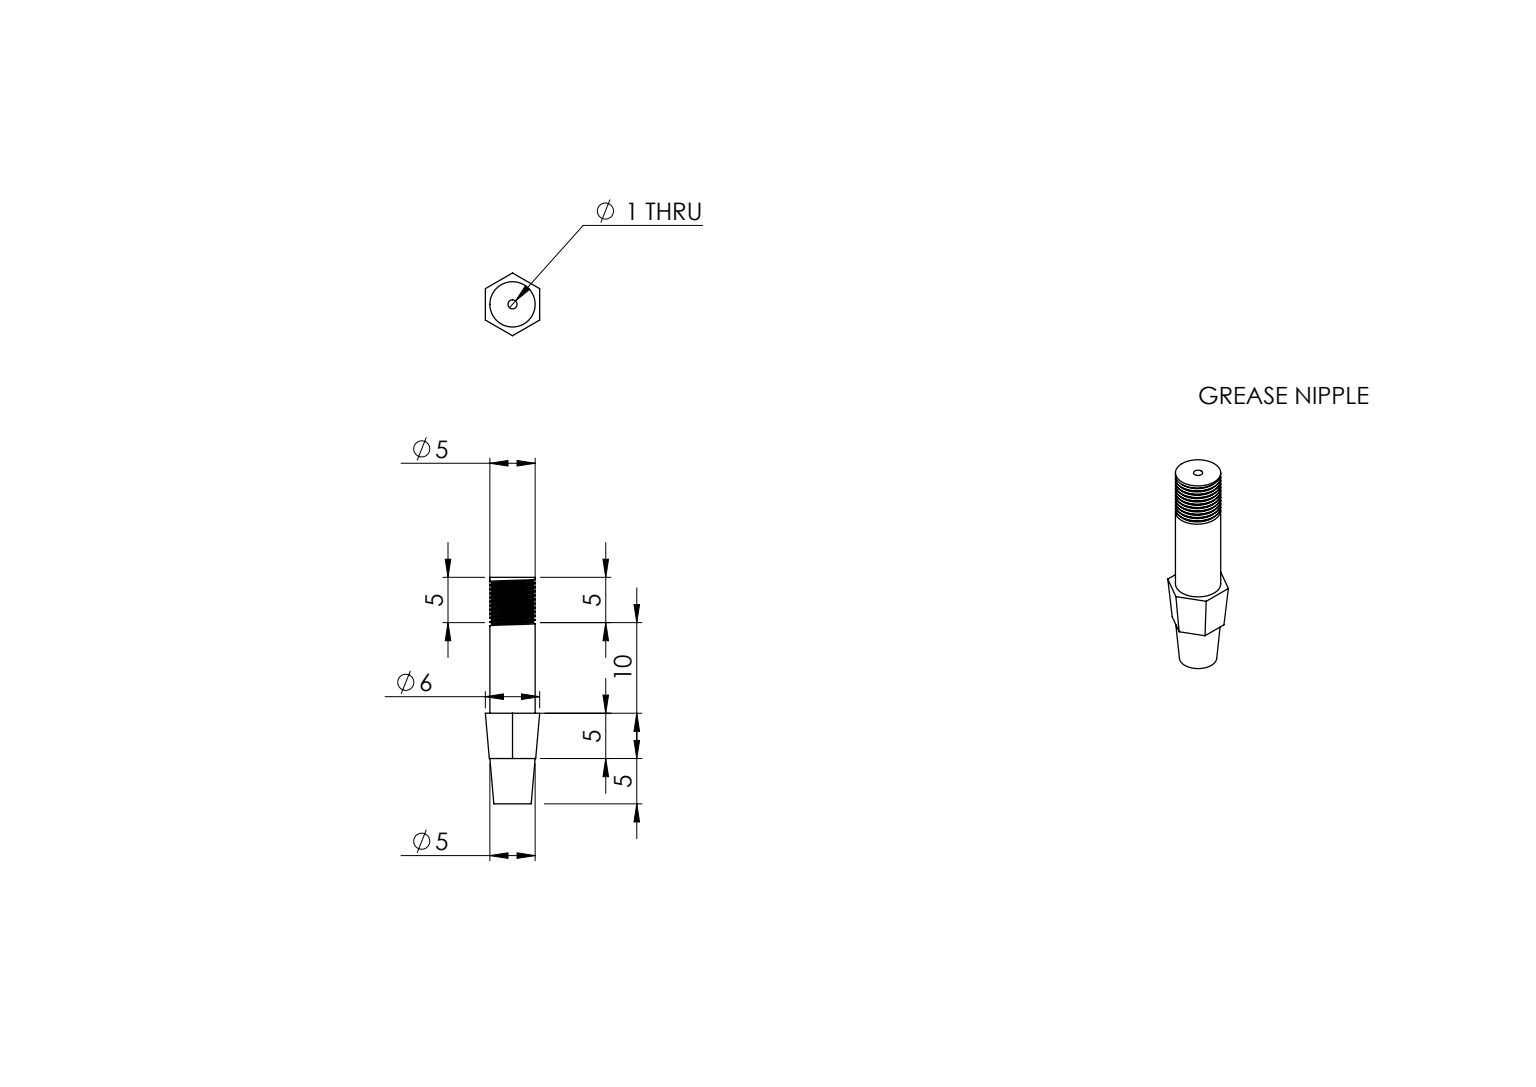
ISO-10303-21;
HEADER;
FILE_DESCRIPTION (('STEP AP214'),
    '1' );
FILE_NAME ('grease nipple.step',
    '2026-10-24T15:06:47',
    ( '' ),
    ( '' ),
    'SwSTEP 2.0',
    'SolidWorks 2026',
    '' );
FILE_SCHEMA (( 'AUTOMOTIVE_DESIGN' ));
ENDSEC;

DATA;
#3=CARTESIAN_POINT ( 'NONE',  ( 4.786228327491940187E-16, -2.728124999385483473, 2.605501347177161087 ) ) ;
#7=CARTESIAN_POINT ( 'NONE',  ( 2.256430356249999658, -2.578124999385483118, -1.302750673588581432 ) ) ;
#11=LINE ( 'NONE', #3942, #5600 ) ;
#16=CARTESIAN_POINT ( 'NONE',  ( 1.128215178125001161, -4.153124999385482852, 1.954126010382870815 ) ) ;
#20=CARTESIAN_POINT ( 'NONE',  ( 1.249999999999999334, -1.050000000000000044, -2.165063509461096825 ) ) ;
#21=CARTESIAN_POINT ( 'NONE',  ( 1.128215178124999607, -3.103124999385482585, -1.954126010382871259 ) ) ;
#25=CARTESIAN_POINT ( 'NONE',  ( 1.250000000000001110, -2.043749998770965970, 2.165063509461096380 ) ) ;
#27=CARTESIAN_POINT ( 'NONE',  ( 1.249999999999999334, -0.9937499987709658145, -2.165063509461096825 ) ) ;
#28=CARTESIAN_POINT ( 'NONE',  ( -2.499999999999999112, -3.112499999999999822, 1.443375672974065882 ) ) ;
#30=CARTESIAN_POINT ( 'NONE',  ( 4.786228327491941173E-16, -3.178124999385482763, 2.605501347177161087 ) ) ;
#31=ORIENTED_EDGE ( 'NONE', *, *, #3987, .F. ) ;
#34=ORIENTED_EDGE ( 'NONE', *, *, #3622, .T. ) ;
#37=CARTESIAN_POINT ( 'NONE',  ( 1.034219503716432668E-14, -3.656249998770965792, -2.500000000000000000 ) ) ;
#40=AXIS2_PLACEMENT_3D ( 'NONE', #3682, #8497, #6028 ) ;
#42=EDGE_CURVE ( 'NONE', #3838, #8637, #9238, .T. ) ;
#46=CARTESIAN_POINT ( 'NONE',  ( -2.256430356249999214, -3.365624999385482319, 1.302750673588581876 ) ) ;
#54=CARTESIAN_POINT ( 'NONE',  ( 3.061616997868383141E-16, 0.000000000000000000, 2.500000000000000000 ) ) ;
#55=CARTESIAN_POINT ( 'NONE',  ( -1.128215178124998497, -3.665624999385482585, 1.954126010382872147 ) ) ;
#57=ORIENTED_EDGE ( 'NONE', *, *, #3072, .T. ) ;
#60=CARTESIAN_POINT ( 'NONE',  ( -2.256430356250000102, -1.940624999385482941, 0.000000000000000000 ) ) ;
#77=CARTESIAN_POINT ( 'NONE',  ( 9.877377282685029372E-16, -1.237499999999999600, 2.500000000000000000 ) ) ;
#78=CARTESIAN_POINT ( 'NONE',  ( 2.256430356250000546, -4.565624999385482496, 1.302750673588579877 ) ) ;
#79=CARTESIAN_POINT ( 'NONE',  ( -4.357666448243394824E-15, -2.531249998770965348, 2.500000000000000000 ) ) ;
#83=CARTESIAN_POINT ( 'NONE',  ( -1.250000000000000222, -4.518749998770965171, -2.165063509461096825 ) ) ;
#88=LINE ( 'NONE', #2497, #4362 ) ;
#89=CARTESIAN_POINT ( 'NONE',  ( 2.256430356249999658, -3.928124999385482319, -1.302750673588581432 ) ) ;
#95=CARTESIAN_POINT ( 'NONE',  ( -2.499999999999999112, -3.506249998770964993, 1.443375672974065882 ) ) ;
#98=ORIENTED_EDGE ( 'NONE', *, *, #7857, .T. ) ;
#99=CARTESIAN_POINT ( 'NONE',  ( 0.000000000000000000, 0.000000000000000000, 0.000000000000000000 ) ) ;
#102=CARTESIAN_POINT ( 'NONE',  ( -2.256430356250000102, -0.1781249993854829572, -1.302750673588580321 ) ) ;
#103=EDGE_CURVE ( 'NONE', #3372, #2494, #7434, .T. ) ;
#104=FACE_OUTER_BOUND ( 'NONE', #9219, .T. ) ;
#110=CARTESIAN_POINT ( 'NONE',  ( -1.128215178124998497, -4.115624999385482319, 1.954126010382872147 ) ) ;
#112=EDGE_LOOP ( 'NONE', ( #9331, #6596, #10060, #487 ) ) ;
#114=CARTESIAN_POINT ( 'NONE',  ( -1.128215178124998497, -3.665624999385482585, 1.954126010382872147 ) ) ;
#121=EDGE_CURVE ( 'NONE', #3756, #7561, #4966, .T. ) ;
#125=ORIENTED_EDGE ( 'NONE', *, *, #7390, .T. ) ;
#127=CARTESIAN_POINT ( 'NONE',  ( 1.250000000000001110, -5.193749998770964993, 2.165063509461096380 ) ) ;
#130=CARTESIAN_POINT ( 'NONE',  ( -2.256430356250000102, -4.303124999385482319, 0.000000000000000000 ) ) ;
#135=CARTESIAN_POINT ( 'NONE',  ( -1.249999999999998224, -4.368749998770964815, 2.165063509461097713 ) ) ;
#138=FACE_OUTER_BOUND ( 'NONE', #6423, .T. ) ;
#141=CARTESIAN_POINT ( 'NONE',  ( -1.128215178125000273, -3.815624999385482941, -1.954126010382871259 ) ) ;
#147=CARTESIAN_POINT ( 'NONE',  ( 1.250000000000001110, -3.843749998770965348, 2.165063509461096380 ) ) ;
#149=EDGE_LOOP ( 'NONE', ( #7106, #3257, #2787, #8826 ) ) ;
#159=CARTESIAN_POINT ( 'NONE',  ( 1.034219503716432668E-14, -4.612500000000000711, -2.500000000000000000 ) ) ;
#160=ORIENTED_EDGE ( 'NONE', *, *, #2379, .T. ) ;
#161=CARTESIAN_POINT ( 'NONE',  ( -2.256430356249999214, -4.153124999385482852, 1.302750673588581876 ) ) ;
#166=CARTESIAN_POINT ( 'NONE',  ( 6.307557144418638510E-17, -20.00000000000000000, -2.958985580760425727 ) ) ;
#167=CARTESIAN_POINT ( 'NONE',  ( 1.250000000000001110, -3.449999999999999289, 2.165063509461096380 ) ) ;
#170=CARTESIAN_POINT ( 'NONE',  ( 1.249999999999999334, -1.443749998770965881, -2.165063509461096825 ) ) ;
#171=CARTESIAN_POINT ( 'NONE',  ( 2.500000000000000000, -4.218749998770966236, -3.061616997868383141E-16 ) ) ;
#172=EDGE_CURVE ( 'NONE', #957, #2983, #5656, .T. ) ;
#173=CARTESIAN_POINT ( 'NONE',  ( -1.128215178125000273, -4.828124999385481786, -1.954126010382871259 ) ) ;
#178=CARTESIAN_POINT ( 'NONE',  ( -1.250000000000000222, -3.618749998770965259, -2.165063509461096825 ) ) ;
#181=EDGE_CURVE ( 'NONE', #471, #3838, #8521, .T. ) ;
#186=CARTESIAN_POINT ( 'NONE',  ( 1.128215178125001161, -4.490624999385482319, 1.954126010382870815 ) ) ;
#191=EDGE_CURVE ( 'NONE', #3656, #1900, #9595, .T. ) ;
#192=PLANE ( 'NONE',  #10324 ) ;
#193=ORIENTED_EDGE ( 'NONE', *, *, #8350, .T. ) ;
#197=CARTESIAN_POINT ( 'NONE',  ( 6.123233995736709336E-17, -25.00000000000000000, 0.4999999999999953371 ) ) ;
#206=CARTESIAN_POINT ( 'NONE',  ( -0.6698729810778081273, -2.157596189432334111, 2.499999999999999112 ) ) ;
#208=CARTESIAN_POINT ( 'NONE',  ( 2.256430356250000546, -4.003124999385482496, 1.302750673588579877 ) ) ;
#211=VECTOR ( 'NONE', #9822, 1000.000000000000000 ) ;
#213=CARTESIAN_POINT ( 'NONE',  ( 2.500000000000000000, -0.6187499987709659255, -3.061616997868383141E-16 ) ) ;
#222=CARTESIAN_POINT ( 'NONE',  ( 2.500000000000000444, -2.456249998770965615, 1.443375672974063439 ) ) ;
#228=CARTESIAN_POINT ( 'NONE',  ( 1.249999999999999334, -5.043749998770965526, -2.165063509461096825 ) ) ;
#230=ORIENTED_EDGE ( 'NONE', *, *, #6289, .F. ) ;
#234=( BOUNDED_CURVE ( )  B_SPLINE_CURVE ( 1, ( #10186, #707 ),
 .UNSPECIFIED., .F., .F. ) 
 B_SPLINE_CURVE_WITH_KNOTS ( ( 2, 2 ),
 ( 0.000000000000000000, 1.000000000000000000 ),
 .UNSPECIFIED. ) 
 CURVE ( )  GEOMETRIC_REPRESENTATION_ITEM ( )  RATIONAL_B_SPLINE_CURVE ( ( 0.9401538480137057174, 0.9401538480137057174 ) ) 
 REPRESENTATION_ITEM ( '' )  );
#238=DIRECTION ( 'NONE',  ( 0.000000000000000000, 0.000000000000000000, -1.000000000000000000 ) ) ;
#239=DIRECTION ( 'NONE',  ( 0.000000000000000000, -1.000000000000000000, 0.000000000000000000 ) ) ;
#253=CARTESIAN_POINT ( 'NONE',  ( -1.250000000000000222, -2.324999999999999734, -2.165063509461096825 ) ) ;
#254=VECTOR ( 'NONE', #2667, 1000.000000000000000 ) ;
#256=CARTESIAN_POINT ( 'NONE',  ( -2.256430356250000546, -5.114265350234221685, -0.8212662131217605133 ) ) ;
#257=SURFACE_STYLE_USAGE ( .BOTH. , #8210 ) ;
#263=ADVANCED_FACE ( 'NONE', ( #4540 ), #1407, .T. ) ;
#270=DIRECTION ( 'NONE',  ( 0.000000000000000000, -1.000000000000000000, 0.000000000000000000 ) ) ;
#273=CARTESIAN_POINT ( 'NONE',  ( 0.000000000000000000, 0.000000000000000000, -2.500000000000000000 ) ) ;
#276=CARTESIAN_POINT ( 'NONE',  ( 4.786228327491941173E-16, -0.5906249993854828517, 2.605501347177161087 ) ) ;
#280=CYLINDRICAL_SURFACE ( 'NONE', #8136, 0.4999999999999953371 ) ;
#287=CARTESIAN_POINT ( 'NONE',  ( 3.061616997868383141E-16, 0.000000000000000000, 2.500000000000000000 ) ) ;
#289=( BOUNDED_CURVE ( )  B_SPLINE_CURVE ( 2, ( #364, #2666, #6794, #9834, #213, #3555, #2617, #5222, #2774 ),
 .UNSPECIFIED., .F., .F. ) 
 B_SPLINE_CURVE_WITH_KNOTS ( ( 3, 2, 2, 2, 3 ),
 ( 0.02083333333333333218, 0.02777777777777777624, 0.04166666666666666435, 0.05555555555555555247, 0.06250000000000000000 ),
 .UNSPECIFIED. ) 
 CURVE ( )  GEOMETRIC_REPRESENTATION_ITEM ( )  RATIONAL_B_SPLINE_CURVE ( ( 0.9330127018922194093, 0.9330127018922194093, 1.000000000000000000, 0.8660254037844387076, 1.000000000000000000, 0.8660254037844387076, 1.000000000000000000, 0.9330127018922194093, 0.9330127018922194093 ) ) 
 REPRESENTATION_ITEM ( '' )  );
#290=ORIENTED_EDGE ( 'NONE', *, *, #2409, .F. ) ;
#293=CARTESIAN_POINT ( 'NONE',  ( -0.6698729810778054627, -2.101346188203299548, 2.500000000000000000 ) ) ;
#308=ORIENTED_EDGE ( 'NONE', *, *, #1549, .F. ) ;
#309=CARTESIAN_POINT ( 'NONE',  ( 5.302876193624534821E-16, -0.3375000000000000222, 2.886751345948128655 ) ) ;
#311=CARTESIAN_POINT ( 'NONE',  ( -2.499999999999999112, -2.662500000000000089, 1.443375672974065882 ) ) ;
#312=CARTESIAN_POINT ( 'NONE',  ( -2.256430356250000102, -0.2906249993854829183, -1.302750673588580321 ) ) ;
#323=CARTESIAN_POINT ( 'NONE',  ( -2.256430356249998770, -5.165624999385483029, 1.302750673588581876 ) ) ;
#329=CARTESIAN_POINT ( 'NONE',  ( -1.128215178124998497, -0.6281249993854828295, 1.954126010382872147 ) ) ;
#338=CARTESIAN_POINT ( 'NONE',  ( 0.000000000000000000, -15.00000000000000000, -3.464101615137755275 ) ) ;
#344=DIRECTION ( 'NONE',  ( 0.000000000000000000, 0.000000000000000000, -1.000000000000000000 ) ) ;
#350=( BOUNDED_CURVE ( )  B_SPLINE_CURVE ( 2, ( #1905, #2558, #5099, #3338, #9762, #1029, #2603, #8299, #3536 ),
 .UNSPECIFIED., .F., .T. ) 
 B_SPLINE_CURVE_WITH_KNOTS ( ( 3, 2, 2, 2, 3 ),
 ( 0.8125000000000000000, 0.8194444444444444198, 0.8333333333333333703, 0.8472222222222222099, 0.8541666666666667407 ),
 .UNSPECIFIED. ) 
 CURVE ( )  GEOMETRIC_REPRESENTATION_ITEM ( )  RATIONAL_B_SPLINE_CURVE ( ( 0.9330127018922194093, 0.9330127018922194093, 1.000000000000000000, 0.8660254037844387076, 1.000000000000000000, 0.8660254037844387076, 1.000000000000000000, 0.9330127018922187432, 0.9330127018922192983 ) ) 
 REPRESENTATION_ITEM ( '' )  );
#352=DIRECTION ( 'NONE',  ( 0.000000000000000000, -1.000000000000000000, 0.000000000000000000 ) ) ;
#353=ADVANCED_FACE ( 'NONE', ( #2833 ), #3833, .T. ) ;
#354=CYLINDRICAL_SURFACE ( 'NONE', #9119, 2.500000000000000000 ) ;
#357=CARTESIAN_POINT ( 'NONE',  ( -2.499999999999999112, -4.856249998770965526, 1.443375672974065882 ) ) ;
#359=CARTESIAN_POINT ( 'NONE',  ( 2.500000000000000000, -2.887500000000000178, -1.443375672974064994 ) ) ;
#364=CARTESIAN_POINT ( 'NONE',  ( -3.486133158594716510E-16, -0.5062499987709657701, -2.500000000000000000 ) ) ;
#372=CARTESIAN_POINT ( 'NONE',  ( 2.256430356250000102, -0.3656249993854829294, -2.763330213280484622E-16 ) ) ;
#381=CARTESIAN_POINT ( 'NONE',  ( 2.256430356250000102, -0.9281249993854827629, -2.763330213280484622E-16 ) ) ;
#384=FACE_OUTER_BOUND ( 'NONE', #8353, .T. ) ;
#386=CARTESIAN_POINT ( 'NONE',  ( -4.357666448243394824E-15, -2.137500000000000178, 2.500000000000000000 ) ) ;
#391=FACE_OUTER_BOUND ( 'NONE', #6159, .T. ) ;
#397=CARTESIAN_POINT ( 'NONE',  ( -3.000000000000000888, -15.00000000000000000, 1.732050807568878525 ) ) ;
#400=EDGE_LOOP ( 'NONE', ( #6468, #2775, #6027, #9450 ) ) ;
#404=CARTESIAN_POINT ( 'NONE',  ( -0.6698729810778054627, -0.3575961894323341772, 2.500000000000000000 ) ) ;
#407=AXIS2_PLACEMENT_3D ( 'NONE', #3351, #3996, #8023 ) ;
#409=EDGE_LOOP ( 'NONE', ( #1063, #2661, #6306, #7148 ) ) ;
#410=CARTESIAN_POINT ( 'NONE',  ( -2.500000000000000000, -0.9375000000000000000, -1.443375672974064106 ) ) ;
#413=CARTESIAN_POINT ( 'NONE',  ( 4.786228327491941173E-16, -0.5906249993854828517, 2.605501347177161087 ) ) ;
#416=ORIENTED_EDGE ( 'NONE', *, *, #4589, .F. ) ;
#418=LINE ( 'NONE', #2620, #6815 ) ;
#425=CARTESIAN_POINT ( 'NONE',  ( 2.256430356250000102, -0.8156249993854828295, -2.763330213280484622E-16 ) ) ;
#433=CARTESIAN_POINT ( 'NONE',  ( 2.256430356250000546, -2.315624999385482496, 1.302750673588579877 ) ) ;
#450=ADVANCED_FACE ( 'NONE', ( #1363 ), #4557, .T. ) ;
#455=CARTESIAN_POINT ( 'NONE',  ( 9.877377282685029372E-16, -0.7312499987709657479, 2.500000000000000000 ) ) ;
#457=CARTESIAN_POINT ( 'NONE',  ( -0.6698729810778069060, -4.086153809338631149, -2.500000000000000000 ) ) ;
#465=CARTESIAN_POINT ( 'NONE',  ( -1.249999999999998224, -1.274999999999999911, 2.165063509461097713 ) ) ;
#468=CARTESIAN_POINT ( 'NONE',  ( -2.256430356249999214, -2.015624999385482674, 1.302750673588581876 ) ) ;
#471=VERTEX_POINT ( 'NONE', #5661 ) ;
#477=CARTESIAN_POINT ( 'NONE',  ( 1.128215178125001161, -0.4406249993854829405, 1.954126010382870815 ) ) ;
#478=CARTESIAN_POINT ( 'NONE',  ( -1.250000000000000222, -4.124999999999999112, -2.165063509461096825 ) ) ;
#480=CARTESIAN_POINT ( 'NONE',  ( 0.6698729810778075722, -1.611153809338631282, 2.499999999999999556 ) ) ;
#487=ORIENTED_EDGE ( 'NONE', *, *, #10255, .F. ) ;
#489=CARTESIAN_POINT ( 'NONE',  ( 2.256430356250000102, -2.278124999385482852, -2.763330213280484622E-16 ) ) ;
#494=CARTESIAN_POINT ( 'NONE',  ( 1.034219503716432668E-14, -4.556249998770965703, -2.500000000000000000 ) ) ;
#502=CARTESIAN_POINT ( 'NONE',  ( 4.996790860652426159E-15, -2.306249998770965259, -2.500000000000000000 ) ) ;
#506=CARTESIAN_POINT ( 'NONE',  ( 2.256430356249999658, -1.228124999385483029, -1.302750673588581432 ) ) ;
#512=EDGE_CURVE ( 'NONE', #9561, #3286, #7220, .T. ) ;
#515=ORIENTED_EDGE ( 'NONE', *, *, #3140, .T. ) ;
#516=ADVANCED_FACE ( 'NONE', ( #8750 ), #3205, .T. ) ;
#520=CARTESIAN_POINT ( 'NONE',  ( 1.250000000000001110, -2.549999999999999822, 2.165063509461096380 ) ) ;
#524=CARTESIAN_POINT ( 'NONE',  ( 1.249999999999999334, -3.750000000000000000, -2.165063509461096825 ) ) ;
#525=CARTESIAN_POINT ( 'NONE',  ( 1.128215178124999607, -0.8531249993854828073, -1.954126010382871259 ) ) ;
#534=CARTESIAN_POINT ( 'NONE',  ( -2.256430356250000102, -1.078124999385482896, -1.302750673588580321 ) ) ;
#545=CARTESIAN_POINT ( 'NONE',  ( 1.128215178125001161, -2.803124999385482319, 1.954126010382870815 ) ) ;
#551=CARTESIAN_POINT ( 'NONE',  ( 1.128215178124999607, -1.303124999385482985, -1.954126010382871259 ) ) ;
#554=CARTESIAN_POINT ( 'NONE',  ( -1.767625397874844694E-16, -0.9562499987709658367, -2.886751345948128655 ) ) ;
#555=DIRECTION ( 'NONE',  ( 0.000000000000000000, 0.000000000000000000, -1.000000000000000000 ) ) ;
#559=CARTESIAN_POINT ( 'NONE',  ( 2.500000000000000444, -4.312499999999999112, 1.443375672974063439 ) ) ;
#560=CARTESIAN_POINT ( 'NONE',  ( -2.256430356250000102, -2.390624999385482674, 0.000000000000000000 ) ) ;
#562=EDGE_CURVE ( 'NONE', #8637, #5955, #6441, .T. ) ;
#571=CARTESIAN_POINT ( 'NONE',  ( -2.500000000000000000, -2.250000000000000000, 0.000000000000000000 ) ) ;
#572=PRODUCT_CONTEXT ( 'NONE', #2270, 'mechanical' ) ;
#575=( BOUNDED_CURVE ( )  B_SPLINE_CURVE ( 2, ( #6071, #8326, #1930, #9321, #2035, #1365, #5230 ),
 .UNSPECIFIED., .F., .F. ) 
 B_SPLINE_CURVE_WITH_KNOTS ( ( 3, 2, 2, 3 ),
 ( 0.8958333333333333703, 0.9027777777777777901, 0.9166666666666666297, 0.9258784757798345089 ),
 .UNSPECIFIED. ) 
 CURVE ( )  GEOMETRIC_REPRESENTATION_ITEM ( )  RATIONAL_B_SPLINE_CURVE ( ( 0.9330127018922192983, 0.9330127018922198534, 1.000000000000000000, 0.8660254037844387076, 1.000000000000000000, 0.9111413147426927761, 0.9401537210011674528 ) ) 
 REPRESENTATION_ITEM ( '' )  );
#576=CARTESIAN_POINT ( 'NONE',  ( -1.595409442497313560E-16, -2.615624999385482319, -2.605501347177161087 ) ) ;
#581=CARTESIAN_POINT ( 'NONE',  ( -2.500000000000000000, -3.131249998770965881, -1.443375672974064106 ) ) ;
#586=CARTESIAN_POINT ( 'NONE',  ( 2.256430356250000546, -0.4031249993854829627, 1.302750673588579877 ) ) ;
#599=CARTESIAN_POINT ( 'NONE',  ( -1.595409442497313560E-16, -4.865624999385482319, -2.605501347177161087 ) ) ;
#602=CARTESIAN_POINT ( 'NONE',  ( 0.6698729810778075722, -0.3174038105676657562, 2.499999999999999556 ) ) ;
#603=AXIS2_PLACEMENT_3D ( 'NONE', #2574, #5908, #1150 ) ;
#604=CARTESIAN_POINT ( 'NONE',  ( 2.256430356250000546, -1.415624999385482807, 1.302750673588579877 ) ) ;
#607=CARTESIAN_POINT ( 'NONE',  ( -2.500000000000000000, -0.3937499987709658922, 0.000000000000000000 ) ) ;
#609=DIRECTION ( 'NONE',  ( 0.8660254037844384856, -0.000000000000000000, 0.5000000000000003331 ) ) ;
#610=LINE ( 'NONE', #5438, #3877 ) ;
#611=CARTESIAN_POINT ( 'NONE',  ( -2.256430356250000102, -1.040624999385483029, 0.000000000000000000 ) ) ;
#617=CARTESIAN_POINT ( 'NONE',  ( -1.250000000000000222, -4.068749998770965881, -2.165063509461096825 ) ) ;
#621=VECTOR ( 'NONE', #847, 1000.000000000000000 ) ;
#625=CARTESIAN_POINT ( 'NONE',  ( -2.500000000000000000, -4.537500000000000533, -1.443375672974064106 ) ) ;
#627=CARTESIAN_POINT ( 'NONE',  ( 1.128215178124999607, -3.103124999385482585, -1.954126010382871259 ) ) ;
#635=CARTESIAN_POINT ( 'NONE',  ( -1.128215178125000273, -0.2156249993854829905, -1.954126010382871259 ) ) ;
#640=CARTESIAN_POINT ( 'NONE',  ( -2.256430356250000102, -2.840624999385482852, 0.000000000000000000 ) ) ;
#641=( BOUNDED_CURVE ( )  B_SPLINE_CURVE ( 2, ( #5478, #4466, #4837, #8031, #171, #6505, #3954, #5728, #2381 ),
 .UNSPECIFIED., .F., .T. ) 
 B_SPLINE_CURVE_WITH_KNOTS ( ( 3, 2, 2, 2, 3 ),
 ( 0.6875000000000000000, 0.6944444444444444198, 0.7083333333333333703, 0.7222222222222222099, 0.7291666666666667407 ),
 .UNSPECIFIED. ) 
 CURVE ( )  GEOMETRIC_REPRESENTATION_ITEM ( )  RATIONAL_B_SPLINE_CURVE ( ( 0.9330127018922194093, 0.9330127018922194093, 1.000000000000000000, 0.8660254037844387076, 1.000000000000000000, 0.8660254037844387076, 1.000000000000000000, 0.9330127018922187432, 0.9330127018922192983 ) ) 
 REPRESENTATION_ITEM ( '' )  );
#652=CARTESIAN_POINT ( 'NONE',  ( 2.256430356250000546, -3.215624999385482408, 1.302750673588579877 ) ) ;
#654=ORIENTED_EDGE ( 'NONE', *, *, #4623, .F. ) ;
#658=CARTESIAN_POINT ( 'NONE',  ( -2.256430356250000102, -2.540624999385482141, -1.302750673588580321 ) ) ;
#660=CARTESIAN_POINT ( 'NONE',  ( 0.000000000000000000, -15.00000000000000000, 0.000000000000000000 ) ) ;
#661=CARTESIAN_POINT ( 'NONE',  ( 2.500000000000000000, -2.381249998770965437, -1.443375672974064994 ) ) ;
#666=CARTESIAN_POINT ( 'NONE',  ( 1.128215178125001161, -0.8906249993854828961, 1.954126010382870815 ) ) ;
#680=CARTESIAN_POINT ( 'NONE',  ( 1.128215178124999607, -1.753124999385482718, -1.954126010382871259 ) ) ;
#687=DIRECTION ( 'NONE',  ( 0.000000000000000000, -1.000000000000000000, 0.000000000000000000 ) ) ;
#689=CARTESIAN_POINT ( 'NONE',  ( 1.128215178124999607, -0.2906249993854829738, -1.954126010382871259 ) ) ;
#690=CARTESIAN_POINT ( 'NONE',  ( 9.877377282685029372E-16, -3.431249998770965259, 2.500000000000000000 ) ) ;
#692=ORIENTED_EDGE ( 'NONE', *, *, #9777, .F. ) ;
#693=CARTESIAN_POINT ( 'NONE',  ( -2.256430356249999214, -1.003124999385482718, 1.302750673588581876 ) ) ;
#702=( BOUNDED_CURVE ( )  B_SPLINE_CURVE ( 2, ( #9940, #9054, #4392, #6590, #2719, #1873, #6743, #7577, #5907 ),
 .UNSPECIFIED., .F., .T. ) 
 B_SPLINE_CURVE_WITH_KNOTS ( ( 3, 2, 2, 2, 3 ),
 ( 0.1458333333333333426, 0.1527777777777777901, 0.1666666666666666574, 0.1805555555555555525, 0.1875000000000000000 ),
 .UNSPECIFIED. ) 
 CURVE ( )  GEOMETRIC_REPRESENTATION_ITEM ( )  RATIONAL_B_SPLINE_CURVE ( ( 0.9330127018922194093, 0.9330127018922194093, 1.000000000000000000, 0.8660254037844387076, 1.000000000000000000, 0.8660254037844387076, 1.000000000000000000, 0.9330127018922194093, 0.9330127018922194093 ) ) 
 REPRESENTATION_ITEM ( '' )  );
#703=CARTESIAN_POINT ( 'NONE',  ( -2.256430356250000102, -4.340624999385482852, -1.302750673588580321 ) ) ;
#705=ADVANCED_FACE ( 'NONE', ( #3545 ), #354, .T. ) ;
#707=CARTESIAN_POINT ( 'NONE',  ( -1.915118561403101438, -5.394273269507307234, -1.606960141313192203 ) ) ;
#708=CARTESIAN_POINT ( 'NONE',  ( -2.256430356250000102, -1.640624999385482896, -1.302750673588580321 ) ) ;
#711=AXIS2_PLACEMENT_3D ( 'NONE', #5088, #4310, #7495 ) ;
#713=CARTESIAN_POINT ( 'NONE',  ( -2.499999999999999556, -2.156249998770965348, 1.443375672974065882 ) ) ;
#716=CARTESIAN_POINT ( 'NONE',  ( -2.500000000000000000, -3.187500000000000000, -1.443375672974064106 ) ) ;
#719=CARTESIAN_POINT ( 'NONE',  ( 1.128215178125001161, -0.4406249993854829405, 1.954126010382870815 ) ) ;
#720=CIRCLE ( 'NONE', #4552, 2.500000000000000444 ) ;
#721=ORIENTED_EDGE ( 'NONE', *, *, #4686, .T. ) ;
#722=EDGE_CURVE ( 'NONE', #8554, #8603, #2756, .T. ) ;
#733=CARTESIAN_POINT ( 'NONE',  ( 2.500000000000000000, -4.237499999999999822, -1.443375672974064994 ) ) ;
#735=CARTESIAN_POINT ( 'NONE',  ( 1.128215178124999607, -4.903124999385481964, -1.954126010382871259 ) ) ;
#736=CARTESIAN_POINT ( 'NONE',  ( 0.000000000000000000, 0.000000000000000000, 0.000000000000000000 ) ) ;
#742=DIRECTION ( 'NONE',  ( -0.08715574274765837404, -0.9961946980917455452, 0.000000000000000000 ) ) ;
#743=CARTESIAN_POINT ( 'NONE',  ( 4.786228327491940187E-16, -4.078124999385482674, 2.605501347177161087 ) ) ;
#747=CARTESIAN_POINT ( 'NONE',  ( -2.256430356249999214, -1.903124999385482852, 1.302750673588581876 ) ) ;
#757=CARTESIAN_POINT ( 'NONE',  ( -2.256430356250000990, -5.226765388979074167, -0.8212675591186288093 ) ) ;
#764=CARTESIAN_POINT ( 'NONE',  ( -1.128215178125000273, -2.578124999385482674, -1.954126010382871259 ) ) ;
#768=CARTESIAN_POINT ( 'NONE',  ( 9.877377282685029372E-16, -1.687499999999999778, 2.500000000000000000 ) ) ;
#769=CARTESIAN_POINT ( 'NONE',  ( -2.499999999999999556, -3.056249998770965259, 1.443375672974065882 ) ) ;
#770=ORIENTED_EDGE ( 'NONE', *, *, #2670, .T. ) ;
#773=CARTESIAN_POINT ( 'NONE',  ( -0.6698729810778020211, -3.242403810567665357, -2.500000000000002665 ) ) ;
#774=FACE_OUTER_BOUND ( 'NONE', #10183, .T. ) ;
#775=CARTESIAN_POINT ( 'NONE',  ( 1.128215178124999607, -3.440624999385482496, -1.954126010382871259 ) ) ;
#778=ORIENTED_EDGE ( 'NONE', *, *, #7478, .F. ) ;
#785=CARTESIAN_POINT ( 'NONE',  ( -1.345399338949505808, -5.026709289312093709, -2.285932919781461958 ) ) ;
#788=CARTESIAN_POINT ( 'NONE',  ( -1.595409442497313560E-16, -4.415624999385482141, -2.605501347177161087 ) ) ;
#791=UNCERTAINTY_MEASURE_WITH_UNIT (LENGTH_MEASURE( 1.000000000000000082E-05 ), #10331, 'distance_accuracy_value', 'NONE');
#799=CARTESIAN_POINT ( 'NONE',  ( -1.595409442497313560E-16, -3.853124999385482585, -2.605501347177161087 ) ) ;
#801=CARTESIAN_POINT ( 'NONE',  ( 2.256430356250000546, -2.203124999385482674, 1.302750673588579877 ) ) ;
#806=CARTESIAN_POINT ( 'NONE',  ( -2.256430356250000102, -0.1406249993854829794, 0.000000000000000000 ) ) ;
#809=CARTESIAN_POINT ( 'NONE',  ( 0.000000000000000000, 0.000000000000000000, 0.000000000000000000 ) ) ;
#815=CARTESIAN_POINT ( 'NONE',  ( 2.256430356249999658, -4.490624999385482319, -1.302750673588581432 ) ) ;
#821=AXIS2_PLACEMENT_3D ( 'NONE', #7498, #239, #4948 ) ;
#822=CARTESIAN_POINT ( 'NONE',  ( 2.500000000000000000, -1.481249998770965970, -1.443375672974064994 ) ) ;
#824=DIRECTION ( 'NONE',  ( 0.000000000000000000, 0.000000000000000000, -1.000000000000000000 ) ) ;
#826=CARTESIAN_POINT ( 'NONE',  ( 2.256430356250000102, -4.415624999385482141, -2.763330213280484622E-16 ) ) ;
#829=CARTESIAN_POINT ( 'NONE',  ( 0.000000000000000000, -25.00000000000000000, -2.062556682370379590 ) ) ;
#830=CARTESIAN_POINT ( 'NONE',  ( 0.000000000000000000, 0.000000000000000000, 0.000000000000000000 ) ) ;
#835=CARTESIAN_POINT ( 'NONE',  ( -1.249999999999998224, -4.875000000000000000, 2.165063509461097713 ) ) ;
#838=CARTESIAN_POINT ( 'NONE',  ( -1.128215178125000273, -3.928124999385483207, -1.954126010382871259 ) ) ;
#843=EDGE_CURVE ( 'NONE', #1838, #1383, #2583, .T. ) ;
#847=DIRECTION ( 'NONE',  ( 0.000000000000000000, -1.000000000000000000, 0.000000000000000000 ) ) ;
#848=CARTESIAN_POINT ( 'NONE',  ( 1.128215178124999607, -3.440624999385482496, -1.954126010382871259 ) ) ;
#850=ADVANCED_FACE ( 'NONE', ( #5431, #7830 ), #2335, .F. ) ;
#852=CARTESIAN_POINT ( 'NONE',  ( 2.256430356250000102, -2.615624999385482763, -2.763330213280484622E-16 ) ) ;
#856=CARTESIAN_POINT ( 'NONE',  ( 1.034219503716432668E-14, -3.206249998770966059, -2.500000000000000000 ) ) ;
#859=( BOUNDED_CURVE ( )  B_SPLINE_CURVE ( 2, ( #959, #2579, #170, #5072, #8963, #4976, #4196, #480, #6128 ),
 .UNSPECIFIED., .F., .F. ) 
 B_SPLINE_CURVE_WITH_KNOTS ( ( 3, 2, 2, 2, 3 ),
 ( 0.1875000000000000000, 0.1944444444444444475, 0.2083333333333333426, 0.2222222222222222099, 0.2291666666666666574 ),
 .UNSPECIFIED. ) 
 CURVE ( )  GEOMETRIC_REPRESENTATION_ITEM ( )  RATIONAL_B_SPLINE_CURVE ( ( 0.9330127018922194093, 0.9330127018922194093, 1.000000000000000000, 0.8660254037844387076, 1.000000000000000000, 0.8660254037844387076, 1.000000000000000000, 0.9330127018922194093, 0.9330127018922194093 ) ) 
 REPRESENTATION_ITEM ( '' )  );
#865=APPLICATION_CONTEXT ( 'automotive_design' ) ;
#867=CARTESIAN_POINT ( 'NONE',  ( 1.128215178125001161, -5.053124999385482319, 1.954126010382870815 ) ) ;
#871=CARTESIAN_POINT ( 'NONE',  ( -1.249999999999998224, -2.568749998770965437, 2.165063509461097713 ) ) ;
#876=CARTESIAN_POINT ( 'NONE',  ( -2.256430356249999214, -3.703124999385482674, 1.302750673588581876 ) ) ;
#880=DIRECTION ( 'NONE',  ( 0.000000000000000000, -1.000000000000000000, 0.000000000000000000 ) ) ;
#883=VECTOR ( 'NONE', #5087, 1000.000000000000114 ) ;
#889=CARTESIAN_POINT ( 'NONE',  ( -1.128215178124998497, -5.128124999385482496, 1.954126010382872147 ) ) ;
#897=CARTESIAN_POINT ( 'NONE',  ( 2.256430356250000546, -3.553124999385482763, 1.302750673588579877 ) ) ;
#899=CARTESIAN_POINT ( 'NONE',  ( 2.256430356250000546, -4.453124999385482674, 1.302750673588579877 ) ) ;
#914=EDGE_CURVE ( 'NONE', #3286, #6080, #4178, .T. ) ;
#916=CARTESIAN_POINT ( 'NONE',  ( 2.256430356250000546, -5.015624999385481786, 1.302750673588579877 ) ) ;
#920=( BOUNDED_CURVE ( )  B_SPLINE_CURVE ( 2, ( #8344, #2554, #4366, #6572, #1021, #8932, #147, #3529, #4218 ),
 .UNSPECIFIED., .F., .T. ) 
 B_SPLINE_CURVE_WITH_KNOTS ( ( 3, 2, 2, 2, 3 ),
 ( 0.6041666666666667407, 0.6111111111111111605, 0.6250000000000000000, 0.6388888888888888395, 0.6458333333333333703 ),
 .UNSPECIFIED. ) 
 CURVE ( )  GEOMETRIC_REPRESENTATION_ITEM ( )  RATIONAL_B_SPLINE_CURVE ( ( 0.9330127018922192983, 0.9330127018922198534, 1.000000000000000000, 0.8660254037844387076, 1.000000000000000000, 0.8660254037844387076, 1.000000000000000000, 0.9330127018922187432, 0.9330127018922192983 ) ) 
 REPRESENTATION_ITEM ( '' )  );
#921=CARTESIAN_POINT ( 'NONE',  ( 2.500000000000000000, -4.631249998770965881, -1.443375672974064994 ) ) ;
#923=CYLINDRICAL_SURFACE ( 'NONE', #5111, 2.500000000000000000 ) ;
#926=CARTESIAN_POINT ( 'NONE',  ( 1.128215178125001161, -4.040624999385483029, 1.954126010382870815 ) ) ;
#929=AXIS2_PLACEMENT_3D ( 'NONE', #6755, #5824, #3568 ) ;
#935=DIRECTION ( 'NONE',  ( 0.000000000000000000, 0.000000000000000000, -1.000000000000000000 ) ) ;
#946=CARTESIAN_POINT ( 'NONE',  ( -2.256430356249998770, -4.153124999385482852, 1.302750673588581876 ) ) ;
#947=ORIENTED_EDGE ( 'NONE', *, *, #3571, .F. ) ;
#948=CARTESIAN_POINT ( 'NONE',  ( -1.595409442497313560E-16, -3.403124999385483296, -2.605501347177161087 ) ) ;
#949=FACE_OUTER_BOUND ( 'NONE', #8574, .T. ) ;
#955=LINE ( 'NONE', #7185, #3544 ) ;
#957=VERTEX_POINT ( 'NONE', #3323 ) ;
#959=CARTESIAN_POINT ( 'NONE',  ( -3.486133158594716510E-16, -1.406249998770965570, -2.500000000000000000 ) ) ;
#962=CARTESIAN_POINT ( 'NONE',  ( -2.256430356249998770, -3.815624999385482941, 1.302750673588581876 ) ) ;
#968=CARTESIAN_POINT ( 'NONE',  ( 2.500000000000000444, -5.156249998770965348, 1.443375672974063439 ) ) ;
#970=ORIENTED_EDGE ( 'NONE', *, *, #3832, .F. ) ;
#971=DIRECTION ( 'NONE',  ( 0.000000000000000000, -1.000000000000000000, 0.000000000000000000 ) ) ;
#974=( BOUNDED_CURVE ( )  B_SPLINE_CURVE ( 2, ( #9222, #7089, #10068, #5429, #4578, #10240, #10294, #2227, #2112, #8722, #4521, #9456, #7714, #1386, #9281, #8618, #6314, #2966, #3849, #2905, #5480, #1442, #7773, #3073, #3126, #4635, #5309, #1542, #551, #2282, #3744, #604, #8504, #7828, #9508, #3901, #3024, #708, #4736, #3802, #6985, #1334, #6927, #10128, #8671, #10187, #6872, #1494, #6200, #6256, #9398, #6145, #9343, #2332, #6089, #2172, #5371, #8561, #4690, #5531, #7930, #658, #764, #7038, #7875, #5580, #2581, #6362, #8869, #4057, #9745, #5774, #4786, #6463, #3956, #4107, #21, #8768, #1784, #3319, #7193, #5731, #9650, #2537, #7983, #5681, #8819, #9556, #6508, #8178, #4980, #7291, #8967, #2384, #3177, #962, #1648, #8917, #1738, #7241, #2488, #3224, #9697, #3361, #1594, #7141, #4935, #6554, #130, #4839, #10346, #4008, #8133, #815, #1694, #78, #4156, #7337, #4891, #8034, #6411, #3271, #173, #8086, #9601, #2433, #5628, #916, #867, #9114, #7430, #323, #8276, #1006, #7483 ),
 .UNSPECIFIED., .F., .T. ) 
 B_SPLINE_CURVE_WITH_KNOTS ( ( 3, 2, 2, 2, 2, 2, 2, 2, 2, 2, 2, 2, 2, 2, 2, 2, 2, 2, 2, 2, 2, 2, 2, 2, 2, 2, 2, 2, 2, 2, 2, 2, 2, 2, 2, 2, 2, 2, 2, 2, 2, 2, 2, 2, 2, 2, 2, 2, 2, 2, 2, 2, 2, 2, 2, 2, 2, 2, 2, 2, 2, 2, 2, 2, 2, 2, 2, 3 ),
 ( 0.000000000000000000, 0.01500076840507158678, 0.03000153681014317356, 0.04500230521521476207, 0.06000307362028634711, 0.07500384202535793909, 0.09000461043042952414, 0.1050053788355011092, 0.1200061472405726942, 0.1350069156456442931, 0.1500076840507158782, 0.1650084524557874632, 0.1800092208608590483, 0.1950099892659306333, 0.2100107576710022184, 0.2250115260760738312, 0.2400122944811453884, 0.2550130628862170012, 0.2700138312912885863, 0.2850145996963601713, 0.3000153681014317564, 0.3150161365065033414, 0.3300169049115749265, 0.3450176733166465115, 0.3600184417217180965, 0.3750192101267896816, 0.3900199785318612666, 0.4050207469369328517, 0.4200215153420044367, 0.4350222837470760773, 0.4500230521521476623, 0.4650238205572192474, 0.4800245889622907769, 0.4950253573673623619, 0.5100261257724340025, 0.5250268941775055875, 0.5400276625825771726, 0.5550284309876486466, 0.5700291993927203427, 0.5850299677977919277, 0.6000307362028635128, 0.6150315046079350978, 0.6300322730130066828, 0.6450330414180782679, 0.6600338098231498529, 0.6750345782282214380, 0.6900353466332930230, 0.7050361150383646081, 0.7200368834434361931, 0.7350376518485077781, 0.7500384202535793632, 0.7650391886586510592, 0.7800399570637225333, 0.7950407254687942293, 0.8100414938738657034, 0.8250422622789372884, 0.8400430306840088734, 0.8550437990890804585, 0.8700445674941521546, 0.8850453358992236286, 0.9000461043042953246, 0.9150468727093667987, 0.9300476411144384947, 0.9450484095195099687, 0.9600491779245815538, 0.9750499463296532499, 0.9900507147347247239, 1.000000000000000000 ),
 .UNSPECIFIED. ) 
 CURVE ( )  GEOMETRIC_REPRESENTATION_ITEM ( )  RATIONAL_B_SPLINE_CURVE ( ( 1.000000000000000000, 0.8660254037844387076, 1.000000000000000000, 0.8660254037844387076, 1.000000000000000000, 0.8660254037844387076, 1.000000000000000000, 0.8660254037844387076, 1.000000000000000000, 0.8660254037844387076, 1.000000000000000000, 0.8660254037844387076, 1.000000000000000000, 0.8660254037844387076, 1.000000000000000000, 0.8660254037844387076, 1.000000000000000000, 0.8660254037844387076, 1.000000000000000000, 0.8660254037844387076, 1.000000000000000000, 0.8660254037844387076, 1.000000000000000000, 0.8660254037844387076, 1.000000000000000000, 0.8660254037844387076, 1.000000000000000000, 0.8660254037844387076, 1.000000000000000000, 0.8660254037844387076, 1.000000000000000000, 0.8660254037844387076, 1.000000000000000000, 0.8660254037844387076, 1.000000000000000000, 0.8660254037844387076, 1.000000000000000000, 0.8660254037844387076, 1.000000000000000000, 0.8660254037844387076, 1.000000000000000000, 0.8660254037844387076, 1.000000000000000000, 0.8660254037844387076, 1.000000000000000000, 0.8660254037844387076, 1.000000000000000000, 0.8660254037844387076, 1.000000000000000000, 0.8660254037844387076, 1.000000000000000000, 0.8660254037844387076, 1.000000000000000000, 0.8660254037844387076, 1.000000000000000000, 0.8660254037844387076, 1.000000000000000000, 0.8660254037844387076, 1.000000000000000000, 0.8660254037844387076, 1.000000000000000000, 0.8660254037844387076, 1.000000000000000000, 0.8660254037844387076, 1.000000000000000000, 0.8660254037844387076, 1.000000000000000000, 0.8660254037844387076, 1.000000000000000000, 0.8660254037844387076, 1.000000000000000000, 0.8660254037844387076, 1.000000000000000000, 0.8660254037844387076, 1.000000000000000000, 0.8660254037844387076, 1.000000000000000000, 0.8660254037844387076, 1.000000000000000000, 0.8660254037844387076, 1.000000000000000000, 0.8660254037844387076, 1.000000000000000000, 0.8660254037844387076, 1.000000000000000000, 0.8660254037844387076, 1.000000000000000000, 0.8660254037844387076, 1.000000000000000000, 0.8660254037844387076, 1.000000000000000000, 0.8660254037844387076, 1.000000000000000000, 0.8660254037844387076, 1.000000000000000000, 0.8660254037844387076, 1.000000000000000000, 0.8660254037844387076, 1.000000000000000000, 0.8660254037844387076, 1.000000000000000000, 0.8660254037844387076, 1.000000000000000000, 0.8660254037844387076, 1.000000000000000000, 0.8660254037844387076, 1.000000000000000000, 0.8660254037844387076, 1.000000000000000000, 0.8660254037844387076, 1.000000000000000000, 0.8660254037844387076, 1.000000000000000000, 0.8660254037844387076, 1.000000000000000000, 0.8660254037844387076, 1.000000000000000000, 0.8660254037844387076, 1.000000000000000000, 0.8660254037844387076, 1.000000000000000000, 0.8660254037844387076, 1.000000000000000000, 0.8660254037844387076, 1.000000000000000000, 0.8660254037844387076, 1.000000000000000000, 0.8660254037844387076, 1.000000000000000000, 0.8660254037844387076, 1.000000000000000000, 0.8660254037844387076, 1.000000000000000000, 0.9111411202376789031, 0.9401538480137057174 ) ) 
 REPRESENTATION_ITEM ( '' )  );
#975=CARTESIAN_POINT ( 'NONE',  ( -2.256430356249999214, -2.803124999385482763, 1.302750673588581876 ) ) ;
#979=CYLINDRICAL_SURFACE ( 'NONE', #821, 2.500000000000000000 ) ;
#986=FACE_OUTER_BOUND ( 'NONE', #5345, .T. ) ;
#987=CARTESIAN_POINT ( 'NONE',  ( 9.877377282685029372E-16, -4.781249998770965348, 2.500000000000000000 ) ) ;
#990=CARTESIAN_POINT ( 'NONE',  ( 2.500000000000000444, -4.762499999999999289, 1.443375672974063439 ) ) ;
#991=ORIENTED_EDGE ( 'NONE', *, *, #6106, .F. ) ;
#992=CARTESIAN_POINT ( 'NONE',  ( -1.128215178124998497, -4.115624999385482319, 1.954126010382872147 ) ) ;
#993=CARTESIAN_POINT ( 'NONE',  ( 1.034219503716432668E-14, -2.812500000000000444, -2.500000000000000000 ) ) ;
#1006=CARTESIAN_POINT ( 'NONE',  ( -2.256430356250000546, -5.226765388979075055, -0.8212675591186288093 ) ) ;
#1012=CARTESIAN_POINT ( 'NONE',  ( -2.499999999999999556, -3.506249998770965437, 1.443375672974065882 ) ) ;
#1013=ORIENTED_EDGE ( 'NONE', *, *, #2364, .F. ) ;
#1018=CARTESIAN_POINT ( 'NONE',  ( 3.486133158594717003E-16, -0.1125000000000000167, -2.500000000000000000 ) ) ;
#1021=CARTESIAN_POINT ( 'NONE',  ( 2.500000000000000000, -3.768749998770965171, -3.061616997868383141E-16 ) ) ;
#1022=( BOUNDED_CURVE ( )  B_SPLINE_CURVE ( 2, ( #9352, #8512, #10138, #8679, #3751, #559, #3135, #7886, #6937 ),
 .UNSPECIFIED., .F., .F. ) 
 B_SPLINE_CURVE_WITH_KNOTS ( ( 3, 2, 2, 2, 3 ),
 ( 0.7708333333333333703, 0.7777777777777777901, 0.7916666666666666297, 0.8055555555555555802, 0.8125000000000000000 ),
 .UNSPECIFIED. ) 
 CURVE ( )  GEOMETRIC_REPRESENTATION_ITEM ( )  RATIONAL_B_SPLINE_CURVE ( ( 0.9330127018922192983, 0.9330127018922198534, 1.000000000000000000, 0.8660254037844387076, 1.000000000000000000, 0.8660254037844387076, 1.000000000000000000, 0.9330127018922194093, 0.9330127018922194093 ) ) 
 REPRESENTATION_ITEM ( '' )  );
#1029=CARTESIAN_POINT ( 'NONE',  ( -2.500000000000000000, -4.537499999999999645, -1.443375672974064106 ) ) ;
#1035=DIRECTION ( 'NONE',  ( 0.000000000000000000, 0.000000000000000000, -1.000000000000000000 ) ) ;
#1041=CARTESIAN_POINT ( 'NONE',  ( -1.128215178124998497, -4.565624999385482496, 1.954126010382872147 ) ) ;
#1042=( LENGTH_UNIT ( ) NAMED_UNIT ( * ) SI_UNIT ( .MILLI., .METRE. ) );
#1062=CARTESIAN_POINT ( 'NONE',  ( 2.256430356249999658, -0.4406249993854829961, -1.302750673588581432 ) ) ;
#1063=ORIENTED_EDGE ( 'NONE', *, *, #7472, .T. ) ;
#1079=AXIS2_PLACEMENT_3D ( 'NONE', #9249, #3872, #6114 ) ;
#1092=CARTESIAN_POINT ( 'NONE',  ( 2.500000000000000000, -0.1875000000000000000, -1.443375672974064994 ) ) ;
#1099=( NAMED_UNIT ( * ) SI_UNIT ( $, .STERADIAN. ) SOLID_ANGLE_UNIT ( ) );
#1103=CARTESIAN_POINT ( 'NONE',  ( 0.000000000000000000, 0.000000000000000000, 0.000000000000000000 ) ) ;
#1113=CARTESIAN_POINT ( 'NONE',  ( -2.500000000000000000, -4.481249998770965526, -1.443375672974064106 ) ) ;
#1115=VECTOR ( 'NONE', #5887, 1000.000000000000000 ) ;
#1122=CARTESIAN_POINT ( 'NONE',  ( -2.500000000000000000, -3.637499999999999734, -1.443375672974064106 ) ) ;
#1128=CARTESIAN_POINT ( 'NONE',  ( -2.499999999999999112, -4.912499999999999645, 1.443375672974065882 ) ) ;
#1134=DIRECTION ( 'NONE',  ( 0.000000000000000000, 0.000000000000000000, -1.000000000000000000 ) ) ;
#1141=CARTESIAN_POINT ( 'NONE',  ( 1.249999999999999334, -4.649999999999999467, -2.165063509461096825 ) ) ;
#1143=CARTESIAN_POINT ( 'NONE',  ( 2.500000000000000000, -1.087500000000000133, -1.443375672974064994 ) ) ;
#1150=DIRECTION ( 'NONE',  ( 0.000000000000000000, 0.000000000000000000, -1.000000000000000000 ) ) ;
#1151=CARTESIAN_POINT ( 'NONE',  ( 1.034219503716432668E-14, -3.206249998770966059, -2.500000000000000000 ) ) ;
#1156=CARTESIAN_POINT ( 'NONE',  ( -2.499999999999999112, -4.012499999999999289, 1.443375672974065882 ) ) ;
#1157=CARTESIAN_POINT ( 'NONE',  ( 9.877377282685029372E-16, -1.181249998770965703, 2.500000000000000000 ) ) ;
#1159=CARTESIAN_POINT ( 'NONE',  ( -0.6698729810778043525, -1.836153809338631593, -2.500000000000001332 ) ) ;
#1163=VERTEX_POINT ( 'NONE', #2953 ) ;
#1165=CARTESIAN_POINT ( 'NONE',  ( -2.256430356250000102, -0.7031249993854828961, 0.000000000000000000 ) ) ;
#1170=CARTESIAN_POINT ( 'NONE',  ( -3.486133158594716510E-16, -3.712499999999999467, -2.500000000000000000 ) ) ;
#1172=( BOUNDED_CURVE ( )  B_SPLINE_CURVE ( 2, ( #6152, #3643, #3808, #5319, #2061, #4525, #8508, #6039, #9349 ),
 .UNSPECIFIED., .F., .F. ) 
 B_SPLINE_CURVE_WITH_KNOTS ( ( 3, 2, 2, 2, 3 ),
 ( 0.5208333333333333703, 0.5277777777777777901, 0.5416666666666666297, 0.5555555555555555802, 0.5625000000000000000 ),
 .UNSPECIFIED. ) 
 CURVE ( )  GEOMETRIC_REPRESENTATION_ITEM ( )  RATIONAL_B_SPLINE_CURVE ( ( 0.9330127018922192983, 0.9330127018922198534, 1.000000000000000000, 0.8660254037844387076, 1.000000000000000000, 0.8660254037844387076, 1.000000000000000000, 0.9330127018922194093, 0.9330127018922194093 ) ) 
 REPRESENTATION_ITEM ( '' )  );
#1177=EDGE_LOOP ( 'NONE', ( #10034, #3325, #6787, #6308, #2950, #2735 ) ) ;
#1181=CARTESIAN_POINT ( 'NONE',  ( 9.877377282685029372E-16, -2.081249998770965615, 2.500000000000000000 ) ) ;
#1192=CARTESIAN_POINT ( 'NONE',  ( -2.500000000000000000, -0.03749999999999999167, -1.443375672974064106 ) ) ;
#1195=CARTESIAN_POINT ( 'NONE',  ( 1.249999999999999334, -1.499999999999999778, -2.165063509461096825 ) ) ;
#1206=CARTESIAN_POINT ( 'NONE',  ( -1.249999999999998224, -3.974999999999999201, 2.165063509461097713 ) ) ;
#1208=CARTESIAN_POINT ( 'NONE',  ( -2.499999999999999112, -1.256249998770965659, 1.443375672974065882 ) ) ;
#1219=CARTESIAN_POINT ( 'NONE',  ( 1.128215178125001161, -1.003124999385482718, 1.954126010382870815 ) ) ;
#1220=ORIENTED_EDGE ( 'NONE', *, *, #7472, .F. ) ;
#1226=ORIENTED_EDGE ( 'NONE', *, *, #4224, .F. ) ;
#1228=DIRECTION ( 'NONE',  ( 0.000000000000000000, -1.000000000000000000, 0.000000000000000000 ) ) ;
#1233=CARTESIAN_POINT ( 'NONE',  ( -2.500000000000000000, -2.193749998770965881, 0.000000000000000000 ) ) ;
#1239=CARTESIAN_POINT ( 'NONE',  ( -3.486133158594716510E-16, -4.106249998770965526, -2.500000000000000000 ) ) ;
#1240=CYLINDRICAL_SURFACE ( 'NONE', #5814, 2.500000000000000000 ) ;
#1242=VERTEX_POINT ( 'NONE', #8712 ) ;
#1246=ORIENTED_EDGE ( 'NONE', *, *, #8836, .T. ) ;
#1247=CARTESIAN_POINT ( 'NONE',  ( 1.250000000000001110, -0.7499999999999998890, 2.165063509461096380 ) ) ;
#1250=CARTESIAN_POINT ( 'NONE',  ( -1.128215178124998497, -1.528124999385482852, 1.954126010382872147 ) ) ;
#1257=VECTOR ( 'NONE', #10093, 1000.000000000000000 ) ;
#1260=VERTEX_POINT ( 'NONE', #3892 ) ;
#1261=CARTESIAN_POINT ( 'NONE',  ( -1.128215178125000273, -2.015624999385483118, -1.954126010382871259 ) ) ;
#1263=EDGE_LOOP ( 'NONE', ( #5643, #8438, #8442, #4121 ) ) ;
#1264=CARTESIAN_POINT ( 'NONE',  ( -1.128215178124998497, -0.9656249993854827407, 1.954126010382872147 ) ) ;
#1269=ORIENTED_EDGE ( 'NONE', *, *, #4456, .T. ) ;
#1271=CARTESIAN_POINT ( 'NONE',  ( -2.256430356250000102, -2.990624999385482763, -1.302750673588580321 ) ) ;
#1272=EDGE_LOOP ( 'NONE', ( #9387, #10151 ) ) ;
#1274=CARTESIAN_POINT ( 'NONE',  ( 1.249999999999999334, -0.5999999999999999778, -2.165063509461096825 ) ) ;
#1275=CARTESIAN_POINT ( 'NONE',  ( 3.486133158594717003E-16, -0.1125000000000000167, -2.500000000000000000 ) ) ;
#1285=CARTESIAN_POINT ( 'NONE',  ( 2.562556682370379146, -20.00000000000000000, 1.479492790380214418 ) ) ;
#1287=CARTESIAN_POINT ( 'NONE',  ( 2.256430356250000546, -2.203124999385482674, 1.302750673588579877 ) ) ;
#1289=ORIENTED_EDGE ( 'NONE', *, *, #9640, .T. ) ;
#1294=ORIENTED_EDGE ( 'NONE', *, *, #8620, .F. ) ;
#1299=CARTESIAN_POINT ( 'NONE',  ( -2.500000000000000000, -1.800000000000000044, 0.000000000000000000 ) ) ;
#1304=CARTESIAN_POINT ( 'NONE',  ( -2.256430356250000102, -2.503124999385482496, 0.000000000000000000 ) ) ;
#1314=CARTESIAN_POINT ( 'NONE',  ( 4.786228327491940187E-16, -0.9281249993854828739, 2.605501347177161087 ) ) ;
#1317=CARTESIAN_POINT ( 'NONE',  ( -2.500000000000000000, -1.331249998770965837, -1.443375672974064106 ) ) ;
#1325=PLANE ( 'NONE',  #40 ) ;
#1326=CARTESIAN_POINT ( 'NONE',  ( 1.128215178125001161, -1.453124999385482896, 1.954126010382870815 ) ) ;
#1334=CARTESIAN_POINT ( 'NONE',  ( 2.256430356249999658, -1.790624999385483029, -1.302750673588581432 ) ) ;
#1337=CARTESIAN_POINT ( 'NONE',  ( -0.6698729810778069060, -2.736153809338631504, -2.500000000000000000 ) ) ;
#1339=EDGE_LOOP ( 'NONE', ( #9519, #2190, #10075, #2428 ) ) ;
#1341=CYLINDRICAL_SURFACE ( 'NONE', #5874, 2.500000000000000000 ) ;
#1342=CARTESIAN_POINT ( 'NONE',  ( 1.128215178124999607, -1.640624999385482896, -1.954126010382871259 ) ) ;
#1344=CARTESIAN_POINT ( 'NONE',  ( 1.045839947578414805E-15, -0.9562499987709659477, -2.500000000000000000 ) ) ;
#1353=CARTESIAN_POINT ( 'NONE',  ( -2.500000000000000000, -1.837499999999999911, -1.443375672974064106 ) ) ;
#1356=CARTESIAN_POINT ( 'NONE',  ( -2.256430356250000102, -2.090624999385482852, -1.302750673588580321 ) ) ;
#1363=FACE_OUTER_BOUND ( 'NONE', #5779, .T. ) ;
#1364=CARTESIAN_POINT ( 'NONE',  ( -2.256430356250000102, -0.5906249993854829627, 0.000000000000000000 ) ) ;
#1365=CARTESIAN_POINT ( 'NONE',  ( -2.499999999999999556, -5.367390331571028739, -0.9099168337232446113 ) ) ;
#1367=PLANE ( 'NONE',  #7746 ) ;
#1368=( BOUNDED_CURVE ( )  B_SPLINE_CURVE ( 2, ( #856, #4047, #7230, #7129, #3262, #6352, #7330, #3353, #10334 ),
 .UNSPECIFIED., .F., .F. ) 
 B_SPLINE_CURVE_WITH_KNOTS ( ( 3, 2, 2, 2, 3 ),
 ( 0.5208333333333333703, 0.5277777777777777901, 0.5416666666666666297, 0.5555555555555555802, 0.5625000000000000000 ),
 .UNSPECIFIED. ) 
 CURVE ( )  GEOMETRIC_REPRESENTATION_ITEM ( )  RATIONAL_B_SPLINE_CURVE ( ( 0.9330127018922192983, 0.9330127018922198534, 1.000000000000000000, 0.8660254037844387076, 1.000000000000000000, 0.8660254037844387076, 1.000000000000000000, 0.9330127018922194093, 0.9330127018922194093 ) ) 
 REPRESENTATION_ITEM ( '' )  );
#1380=VERTEX_POINT ( 'NONE', #8758 ) ;
#1381=CARTESIAN_POINT ( 'NONE',  ( 2.256430356250000102, -4.978124999385482141, -2.763330213280484622E-16 ) ) ;
#1383=VERTEX_POINT ( 'NONE', #7971 ) ;
#1385=CARTESIAN_POINT ( 'NONE',  ( 2.500000000000000444, -0.2625000000000000111, 1.443375672974063439 ) ) ;
#1386=CARTESIAN_POINT ( 'NONE',  ( -2.256430356250000102, -0.7406249993854829849, -1.302750673588580321 ) ) ;
#1394=CARTESIAN_POINT ( 'NONE',  ( -0.2187216588148106211, -20.00000000000000000, -3.085264589354758336 ) ) ;
#1395=ORIENTED_EDGE ( 'NONE', *, *, #843, .T. ) ;
#1398=CARTESIAN_POINT ( 'NONE',  ( 2.256430356249999658, -1.678124999385482541, -1.302750673588581432 ) ) ;
#1400=DIRECTION ( 'NONE',  ( -0.000000000000000000, -1.000000000000000000, -0.000000000000000000 ) ) ;
#1405=ORIENTED_EDGE ( 'NONE', *, *, #1450, .F. ) ;
#1407=CYLINDRICAL_SURFACE ( 'NONE', #5293, 2.500000000000000000 ) ;
#1409=CARTESIAN_POINT ( 'NONE',  ( 2.500000000000000444, -2.962499999999999467, 1.443375672974063439 ) ) ;
#1410=CARTESIAN_POINT ( 'NONE',  ( 1.045839947578414805E-15, -0.9562499987709659477, -2.500000000000000000 ) ) ;
#1411=CARTESIAN_POINT ( 'NONE',  ( -2.256430356249999214, -2.915624999385482585, 1.302750673588581876 ) ) ;
#1424=CARTESIAN_POINT ( 'NONE',  ( 1.128215178125001161, -1.340624999385482852, 1.954126010382870815 ) ) ;
#1427=CARTESIAN_POINT ( 'NONE',  ( 1.128215178125001161, -2.690624999385482941, 1.954126010382870815 ) ) ;
#1437=CARTESIAN_POINT ( 'NONE',  ( -1.595409442497313560E-16, -3.965624999385482408, -2.605501347177161087 ) ) ;
#1439=ORIENTED_EDGE ( 'NONE', *, *, #4589, .T. ) ;
#1442=CARTESIAN_POINT ( 'NONE',  ( 4.786228327491940187E-16, -1.040624999385482807, 2.605501347177161087 ) ) ;
#1444=VERTEX_POINT ( 'NONE', #1687 ) ;
#1446=CARTESIAN_POINT ( 'NONE',  ( 1.249999999999999334, -2.793749998770965526, -2.165063509461096825 ) ) ;
#1450=EDGE_CURVE ( 'NONE', #6810, #8910, #1368, .T. ) ;
#1452=CARTESIAN_POINT ( 'NONE',  ( 4.786228327491941173E-16, -1.378124999385482941, 2.605501347177161087 ) ) ;
#1459=CARTESIAN_POINT ( 'NONE',  ( -0.6698729810778020211, -3.636153809338631415, -2.500000000000002665 ) ) ;
#1460=ORIENTED_EDGE ( 'NONE', *, *, #3571, .T. ) ;
#1462=VECTOR ( 'NONE', #7270, 1000.000000000000000 ) ;
#1464=CARTESIAN_POINT ( 'NONE',  ( 2.500000000000000444, -3.412500000000000089, 1.443375672974063439 ) ) ;
#1467=CARTESIAN_POINT ( 'NONE',  ( 1.128215178125001161, -1.453124999385482896, 1.954126010382870815 ) ) ;
#1471=CARTESIAN_POINT ( 'NONE',  ( 1.250000000000001110, -2.100000000000000089, 2.165063509461096380 ) ) ;
#1474=CARTESIAN_POINT ( 'NONE',  ( 2.256430356250000546, -0.8531249993854829183, 1.302750673588579877 ) ) ;
#1478=CARTESIAN_POINT ( 'NONE',  ( -1.128215178125000273, -1.115624999385482985, -1.954126010382871259 ) ) ;
#1488=EDGE_LOOP ( 'NONE', ( #2508, #3884 ) ) ;
#1489=CARTESIAN_POINT ( 'NONE',  ( 1.128215178125001161, -5.053124999385482319, 1.954126010382870815 ) ) ;
#1494=CARTESIAN_POINT ( 'NONE',  ( -2.256430356249998770, -2.015624999385482674, 1.302750673588581876 ) ) ;
#1498=CARTESIAN_POINT ( 'NONE',  ( -1.250000000000000222, -2.718749998770965792, -2.165063509461096825 ) ) ;
#1501=ORIENTED_EDGE ( 'NONE', *, *, #10290, .F. ) ;
#1502=CARTESIAN_POINT ( 'NONE',  ( 0.000000000000000000, 0.000000000000000000, 0.000000000000000000 ) ) ;
#1503=CARTESIAN_POINT ( 'NONE',  ( -1.595409442497313560E-16, -2.053124999385482763, -2.605501347177161087 ) ) ;
#1507=DIRECTION ( 'NONE',  ( 0.000000000000000000, -1.000000000000000000, 0.000000000000000000 ) ) ;
#1508=CARTESIAN_POINT ( 'NONE',  ( 9.877377282685029372E-16, -3.431249998770965259, 2.500000000000000000 ) ) ;
#1513=CARTESIAN_POINT ( 'NONE',  ( 2.500000000000000000, -3.824999999999999734, -3.061616997868383141E-16 ) ) ;
#1516=CARTESIAN_POINT ( 'NONE',  ( -1.128215178124998497, -4.678124999385482319, 1.954126010382872147 ) ) ;
#1522=EDGE_CURVE ( 'NONE', #7872, #10235, #289, .T. ) ;
#1524=CARTESIAN_POINT ( 'NONE',  ( -1.128215178124998497, -3.215624999385482408, 1.954126010382872147 ) ) ;
#1527=CARTESIAN_POINT ( 'NONE',  ( 2.256430356249999658, -3.028124999385482852, -1.302750673588581432 ) ) ;
#1532=DIRECTION ( 'NONE',  ( 0.000000000000000000, -1.000000000000000000, 0.000000000000000000 ) ) ;
#1535=CARTESIAN_POINT ( 'NONE',  ( -2.256430356249999214, -5.165624999385481253, 1.302750673588581876 ) ) ;
#1541=CARTESIAN_POINT ( 'NONE',  ( 2.500000000000000000, -1.125000000000000000, -3.061616997868383141E-16 ) ) ;
#1542=CARTESIAN_POINT ( 'NONE',  ( -1.595409442497313560E-16, -1.265624999385482896, -2.605501347177161087 ) ) ;
#1543=CARTESIAN_POINT ( 'NONE',  ( -2.562556682370380035, -20.00000000000000000, -1.479492790380212641 ) ) ;
#1549=EDGE_CURVE ( 'NONE', #4027, #4436, #702, .T. ) ;
#1551=CARTESIAN_POINT ( 'NONE',  ( 2.500000000000000000, -1.968749998770965792, -3.061616997868383141E-16 ) ) ;
#1552=CARTESIAN_POINT ( 'NONE',  ( 2.500000000000000444, -1.106249998770965748, 1.443375672974063439 ) ) ;
#1553=CARTESIAN_POINT ( 'NONE',  ( -1.249999999999998224, -3.074999999999999734, 2.165063509461097713 ) ) ;
#1555=CARTESIAN_POINT ( 'NONE',  ( -1.128215178124998497, -4.565624999385482496, 1.954126010382872147 ) ) ;
#1564=CARTESIAN_POINT ( 'NONE',  ( 1.250000000000001110, -4.799999999999999822, 2.165063509461096380 ) ) ;
#1567=CARTESIAN_POINT ( 'NONE',  ( -1.128215178124998497, -3.328124999385482230, 1.954126010382872147 ) ) ;
#1572=CARTESIAN_POINT ( 'NONE',  ( 2.562556682370379146, -20.00000000000000000, -1.479492790380211975 ) ) ;
#1575=CARTESIAN_POINT ( 'NONE',  ( 1.128215178125001161, -4.040624999385483029, 1.954126010382870815 ) ) ;
#1577=CARTESIAN_POINT ( 'NONE',  ( -2.256430356250000102, -3.290624999385482585, 0.000000000000000000 ) ) ;
#1583=ORIENTED_EDGE ( 'NONE', *, *, #4726, .F. ) ;
#1587=ORIENTED_EDGE ( 'NONE', *, *, #6647, .T. ) ;
#1588=CARTESIAN_POINT ( 'NONE',  ( 1.128215178124999607, -3.553124999385482319, -1.954126010382871259 ) ) ;
#1594=CARTESIAN_POINT ( 'NONE',  ( 1.128215178125001161, -4.153124999385482852, 1.954126010382870815 ) ) ;
#1600=CARTESIAN_POINT ( 'NONE',  ( 2.500000000000000000, -2.418749998770965526, -3.061616997868383141E-16 ) ) ;
#1602=DIRECTION ( 'NONE',  ( -0.8660254037844387076, 0.000000000000000000, 0.4999999999999997780 ) ) ;
#1605=CARTESIAN_POINT ( 'NONE',  ( 2.256430356249999658, -4.378124999385482496, -1.302750673588581432 ) ) ;
#1610=CARTESIAN_POINT ( 'NONE',  ( 2.500000000000000444, -2.006249998770965437, 1.443375672974063439 ) ) ;
#1614=CARTESIAN_POINT ( 'NONE',  ( -2.500000000000000000, -4.500000000000000000, 0.000000000000000000 ) ) ;
#1618=CARTESIAN_POINT ( 'NONE',  ( 2.256430356250000546, -4.115624999385482319, 1.302750673588579877 ) ) ;
#1623=CLOSED_SHELL ( 'NONE', ( #5370, #3449, #10043, #5707, #9961, #3096, #3479, #7749, #3029, #8381, #5143, #705, #2732, #8657, #7497, #4346, #6568, #450, #263, #3444, #7268, #353, #7296, #4321, #7841, #5938, #9422, #2541, #516, #9883, #8829, #8223, #6008, #5300, #850, #6187, #1655, #8598, #9908, #4619, #9910, #1766, #7827 ) ) ;
#1628=CARTESIAN_POINT ( 'NONE',  ( -1.128215178124998497, -2.765624999385482674, 1.954126010382872147 ) ) ;
#1630=EDGE_LOOP ( 'NONE', ( #3710, #125, #4256, #778 ) ) ;
#1632=CARTESIAN_POINT ( 'NONE',  ( -1.128215178125000273, -3.365624999385482763, -1.954126010382871259 ) ) ;
#1637=CARTESIAN_POINT ( 'NONE',  ( 3.000000000000000000, -15.00000000000000000, 1.732050807568879192 ) ) ;
#1648=CARTESIAN_POINT ( 'NONE',  ( -2.256430356250000102, -3.853124999385482585, 0.000000000000000000 ) ) ;
#1651=( BOUNDED_CURVE ( )  B_SPLINE_CURVE ( 2, ( #1508, #5545, #8636, #95, #3920, #7205, #9522, #1459, #37 ),
 .UNSPECIFIED., .F., .F. ) 
 B_SPLINE_CURVE_WITH_KNOTS ( ( 3, 2, 2, 2, 3 ),
 ( 0.5625000000000000000, 0.5694444444444444198, 0.5833333333333333703, 0.5972222222222222099, 0.6041666666666667407 ),
 .UNSPECIFIED. ) 
 CURVE ( )  GEOMETRIC_REPRESENTATION_ITEM ( )  RATIONAL_B_SPLINE_CURVE ( ( 0.9330127018922194093, 0.9330127018922194093, 1.000000000000000000, 0.8660254037844387076, 1.000000000000000000, 0.8660254037844387076, 1.000000000000000000, 0.9330127018922187432, 0.9330127018922192983 ) ) 
 REPRESENTATION_ITEM ( '' )  );
#1654=CARTESIAN_POINT ( 'NONE',  ( -1.767625397874844694E-16, -1.856249998770965526, -2.886751345948128655 ) ) ;
#1655=ADVANCED_FACE ( 'NONE', ( #2813, #3864 ), #10084, .T. ) ;
#1657=FACE_BOUND ( 'NONE', #8386, .T. ) ;
#1659=CARTESIAN_POINT ( 'NONE',  ( -1.595409442497313560E-16, -4.303124999385482319, -2.605501347177161087 ) ) ;
#1663=CARTESIAN_POINT ( 'NONE',  ( -9.703070624755296135E-15, -3.487499999999999822, 2.500000000000000444 ) ) ;
#1670=CARTESIAN_POINT ( 'NONE',  ( 2.256430356249999658, -4.940624999385482496, -1.302750673588581432 ) ) ;
#1680=CARTESIAN_POINT ( 'NONE',  ( 4.786228327491940187E-16, -3.178124999385483207, 2.605501347177161087 ) ) ;
#1683=CARTESIAN_POINT ( 'NONE',  ( -2.500000000000000000, -0.4874999999999999334, -1.443375672974064106 ) ) ;
#1687=CARTESIAN_POINT ( 'NONE',  ( -1.915118561403101438, -5.394273269507307234, -1.606960141313192203 ) ) ;
#1693=CARTESIAN_POINT ( 'NONE',  ( 0.6698729810778063509, -1.032596189432334111, -2.500000000000000000 ) ) ;
#1694=CARTESIAN_POINT ( 'NONE',  ( 2.256430356250000102, -4.528124999385481964, -2.763330213280484622E-16 ) ) ;
#1698=CARTESIAN_POINT ( 'NONE',  ( 2.500000000000000444, -4.256249998770965881, 1.443375672974063439 ) ) ;
#1702=CARTESIAN_POINT ( 'NONE',  ( -2.500000000000000000, 0.000000000000000000, 0.000000000000000000 ) ) ;
#1703=CARTESIAN_POINT ( 'NONE',  ( 2.256430356250000102, -3.515624999385482674, -2.763330213280484622E-16 ) ) ;
#1705=EDGE_CURVE ( 'NONE', #7134, #10177, #7370, .T. ) ;
#1706=ORIENTED_EDGE ( 'NONE', *, *, #8873, .T. ) ;
#1712=AXIS2_PLACEMENT_3D ( 'NONE', #3630, #6920, #6811 ) ;
#1715=CARTESIAN_POINT ( 'NONE',  ( -1.595409442497313560E-16, -0.2531249993854829405, -2.605501347177161087 ) ) ;
#1726=CARTESIAN_POINT ( 'NONE',  ( 2.256430356249999658, -2.578124999385483118, -1.302750673588581432 ) ) ;
#1728=CARTESIAN_POINT ( 'NONE',  ( -1.595409442497313560E-16, -3.853124999385482585, -2.605501347177161087 ) ) ;
#1738=CARTESIAN_POINT ( 'NONE',  ( -1.128215178125000273, -3.928124999385483207, -1.954126010382871259 ) ) ;
#1742=CARTESIAN_POINT ( 'NONE',  ( 1.250000000000001110, -5.193749998770964993, 2.165063509461096380 ) ) ;
#1745=CARTESIAN_POINT ( 'NONE',  ( 0.000000000000000000, 0.000000000000000000, -2.500000000000000000 ) ) ;
#1748=CARTESIAN_POINT ( 'NONE',  ( -1.128215178124998497, -5.015624999385482674, 1.954126010382872147 ) ) ;
#1751=CARTESIAN_POINT ( 'NONE',  ( -0.6698729810778069060, -3.692403810567665978, -2.500000000000000000 ) ) ;
#1754=( BOUNDED_CURVE ( )  B_SPLINE_CURVE ( 2, ( #5225, #4498, #7691, #6904, #2146, #10099, #1471, #4868, #9629 ),
 .UNSPECIFIED., .F., .T. ) 
 B_SPLINE_CURVE_WITH_KNOTS ( ( 3, 2, 2, 2, 3 ),
 ( 0.3541666666666666852, 0.3611111111111111049, 0.3750000000000000000, 0.3888888888888888951, 0.3958333333333333703 ),
 .UNSPECIFIED. ) 
 CURVE ( )  GEOMETRIC_REPRESENTATION_ITEM ( )  RATIONAL_B_SPLINE_CURVE ( ( 0.9330127018922194093, 0.9330127018922196314, 1.000000000000000000, 0.8660254037844387076, 1.000000000000000000, 0.8660254037844387076, 1.000000000000000000, 0.9330127018922190762, 0.9330127018922194093 ) ) 
 REPRESENTATION_ITEM ( '' )  );
#1766=ADVANCED_FACE ( 'NONE', ( #1922 ), #5239, .T. ) ;
#1768=CARTESIAN_POINT ( 'NONE',  ( 2.256430356250000546, -4.903124999385481964, 1.302750673588579877 ) ) ;
#1784=CARTESIAN_POINT ( 'NONE',  ( 2.256430356250000102, -3.178124999385482319, -2.763330213280484622E-16 ) ) ;
#1785=CARTESIAN_POINT ( 'NONE',  ( 0.6698729810778087934, -2.326346188203300525, -2.499999999999999112 ) ) ;
#1787=CARTESIAN_POINT ( 'NONE',  ( -0.6698729810778043525, -1.892403810567665712, -2.500000000000001332 ) ) ;
#1788=ORIENTED_EDGE ( 'NONE', *, *, #3153, .T. ) ;
#1789=CARTESIAN_POINT ( 'NONE',  ( 2.500000000000000000, -3.731249998770965970, -1.443375672974064994 ) ) ;
#1798=ORIENTED_EDGE ( 'NONE', *, *, #3264, .T. ) ;
#1799=CIRCLE ( 'NONE', #7161, 2.500000000000000000 ) ;
#1808=VERTEX_POINT ( 'NONE', #1170 ) ;
#1815=CARTESIAN_POINT ( 'NONE',  ( 0.000000000000000000, -25.00000000000000000, 0.000000000000000000 ) ) ;
#1817=CARTESIAN_POINT ( 'NONE',  ( 4.786228327491941173E-16, -4.978124999385483029, 2.605501347177161087 ) ) ;
#1823=EDGE_CURVE ( 'NONE', #8910, #4703, #4211, .T. ) ;
#1824=CARTESIAN_POINT ( 'NONE',  ( -1.250000000000000222, -1.424999999999999822, -2.165063509461096825 ) ) ;
#1836=CARTESIAN_POINT ( 'NONE',  ( -2.256430356250000102, -0.2906249993854829183, -1.302750673588580321 ) ) ;
#1838=VERTEX_POINT ( 'NONE', #2692 ) ;
#1842=DIRECTION ( 'NONE',  ( 0.000000000000000000, -1.000000000000000000, 0.000000000000000000 ) ) ;
#1844=EDGE_CURVE ( 'NONE', #8603, #3561, #8215, .T. ) ;
#1848=CARTESIAN_POINT ( 'NONE',  ( -4.357666448243394824E-15, -2.587499999999999467, 2.500000000000000000 ) ) ;
#1863=CARTESIAN_POINT ( 'NONE',  ( -3.486133158594716510E-16, -0.5062499987709657701, -2.500000000000000000 ) ) ;
#1866=CARTESIAN_POINT ( 'NONE',  ( 1.249999999999999334, -0.1499999999999999944, -2.165063509461096825 ) ) ;
#1873=CARTESIAN_POINT ( 'NONE',  ( -2.500000000000000000, -0.9375000000000000000, -1.443375672974064106 ) ) ;
#1881=CARTESIAN_POINT ( 'NONE',  ( -2.500000000000000000, -1.743749998770965925, 0.000000000000000000 ) ) ;
#1882=CARTESIAN_POINT ( 'NONE',  ( 1.250000000000001110, -2.493749998770965703, 2.165063509461096380 ) ) ;
#1887=CARTESIAN_POINT ( 'NONE',  ( -2.500000000000000000, -4.031249998770966236, -1.443375672974064106 ) ) ;
#1888=ORIENTED_EDGE ( 'NONE', *, *, #722, .T. ) ;
#1895=( BOUNDED_CURVE ( )  B_SPLINE_CURVE ( 2, ( #8730, #6369, #1553, #28, #7939, #716, #5690, #773, #4899 ),
 .UNSPECIFIED., .F., .F. ) 
 B_SPLINE_CURVE_WITH_KNOTS ( ( 3, 2, 2, 2, 3 ),
 ( 0.5625000000000000000, 0.5694444444444444198, 0.5833333333333333703, 0.5972222222222222099, 0.6041666666666667407 ),
 .UNSPECIFIED. ) 
 CURVE ( )  GEOMETRIC_REPRESENTATION_ITEM ( )  RATIONAL_B_SPLINE_CURVE ( ( 0.9330127018922194093, 0.9330127018922194093, 1.000000000000000000, 0.8660254037844387076, 1.000000000000000000, 0.8660254037844387076, 1.000000000000000000, 0.9330127018922187432, 0.9330127018922192983 ) ) 
 REPRESENTATION_ITEM ( '' )  );
#1900=VERTEX_POINT ( 'NONE', #1018 ) ;
#1902=CYLINDRICAL_SURFACE ( 'NONE', #3076, 2.500000000000000000 ) ;
#1905=CARTESIAN_POINT ( 'NONE',  ( 9.877377282685029372E-16, -4.387499999999999289, 2.500000000000000000 ) ) ;
#1911=DIRECTION ( 'NONE',  ( 0.000000000000000000, -1.000000000000000000, 0.000000000000000000 ) ) ;
#1912=CARTESIAN_POINT ( 'NONE',  ( 1.034219503716432668E-14, -4.556249998770965703, -2.500000000000000000 ) ) ;
#1915=DIRECTION ( 'NONE',  ( 0.000000000000000000, 0.000000000000000000, -1.000000000000000000 ) ) ;
#1916=CARTESIAN_POINT ( 'NONE',  ( -2.256430356250000102, -5.090624999385482852, 0.000000000000000000 ) ) ;
#1918=EDGE_CURVE ( 'NONE', #1242, #2167, #10129, .T. ) ;
#1919=CARTESIAN_POINT ( 'NONE',  ( 1.249999999999999334, -2.849999999999999645, -2.165063509461096825 ) ) ;
#1922=FACE_OUTER_BOUND ( 'NONE', #6392, .T. ) ;
#1925=CARTESIAN_POINT ( 'NONE',  ( 3.061616997868383141E-16, 0.000000000000000000, 2.500000000000000000 ) ) ;
#1930=CARTESIAN_POINT ( 'NONE',  ( -1.249999999999998224, -5.268749998770966059, 2.165063509461097713 ) ) ;
#1941=CARTESIAN_POINT ( 'NONE',  ( -2.256430356249999214, -1.115624999385482763, 1.302750673588581876 ) ) ;
#1947=STYLED_ITEM ( 'NONE', ( #7417 ), #5870 ) ;
#1951=CARTESIAN_POINT ( 'NONE',  ( -1.249999999999998224, -0.7687499987709658367, 2.165063509461097713 ) ) ;
#1962=( BOUNDED_CURVE ( )  B_SPLINE_CURVE ( 2, ( #6014, #10045, #2883, #3049, #7855, #581, #5459, #6961, #6066 ),
 .UNSPECIFIED., .F., .F. ) 
 B_SPLINE_CURVE_WITH_KNOTS ( ( 3, 2, 2, 2, 3 ),
 ( 0.4791666666666666852, 0.4861111111111111049, 0.5000000000000000000, 0.5138888888888888395, 0.5208333333333333703 ),
 .UNSPECIFIED. ) 
 CURVE ( )  GEOMETRIC_REPRESENTATION_ITEM ( )  RATIONAL_B_SPLINE_CURVE ( ( 0.9330127018922194093, 0.9330127018922196314, 1.000000000000000000, 0.8660254037844387076, 1.000000000000000000, 0.8660254037844387076, 1.000000000000000000, 0.9330127018922187432, 0.9330127018922192983 ) ) 
 REPRESENTATION_ITEM ( '' )  );
#1967=CARTESIAN_POINT ( 'NONE',  ( -2.500000000000000000, 0.000000000000000000, 0.000000000000000000 ) ) ;
#1968=VERTEX_POINT ( 'NONE', #4468 ) ;
#1969=CARTESIAN_POINT ( 'NONE',  ( 5.302876193624534821E-16, -1.237499999999999822, 2.886751345948128655 ) ) ;
#1971=CARTESIAN_POINT ( 'NONE',  ( -1.250000000000000222, -2.774999999999999467, -2.165063509461096825 ) ) ;
#1978=CARTESIAN_POINT ( 'NONE',  ( -1.249999999999998224, -1.274999999999999911, 2.165063509461097713 ) ) ;
#1983=ORIENTED_EDGE ( 'NONE', *, *, #172, .F. ) ;
#1984=FACE_OUTER_BOUND ( 'NONE', #10327, .T. ) ;
#1989=EDGE_LOOP ( 'NONE', ( #6193, #2273, #7966, #5164 ) ) ;
#1991=CARTESIAN_POINT ( 'NONE',  ( 1.128215178124999607, -2.203124999385482674, -1.954126010382871259 ) ) ;
#1994=CARTESIAN_POINT ( 'NONE',  ( 2.500000000000000000, -0.6749999999999999334, -3.061616997868383141E-16 ) ) ;
#1997=EDGE_LOOP ( 'NONE', ( #7091, #7609, #5760, #4747 ) ) ;
#1998=CARTESIAN_POINT ( 'NONE',  ( -1.250000000000000222, -0.4687499987709658478, -2.165063509461096825 ) ) ;
#2007=EDGE_LOOP ( 'NONE', ( #8523, #10020, #4656, #6965 ) ) ;
#2020=CARTESIAN_POINT ( 'NONE',  ( -1.249999999999998224, -2.174999999999999822, 2.165063509461097713 ) ) ;
#2023=LINE ( 'NONE', #9990, #1257 ) ;
#2024=( BOUNDED_CURVE ( )  B_SPLINE_CURVE ( 2, ( #3510, #5182, #2839, #5867, #1881, #7533, #3462, #1159, #2677 ),
 .UNSPECIFIED., .F., .T. ) 
 B_SPLINE_CURVE_WITH_KNOTS ( ( 3, 2, 2, 2, 3 ),
 ( 0.2291666666666666574, 0.2361111111111111049, 0.2500000000000000000, 0.2638888888888888951, 0.2708333333333333703 ),
 .UNSPECIFIED. ) 
 CURVE ( )  GEOMETRIC_REPRESENTATION_ITEM ( )  RATIONAL_B_SPLINE_CURVE ( ( 0.9330127018922194093, 0.9330127018922194093, 1.000000000000000000, 0.8660254037844387076, 1.000000000000000000, 0.8660254037844387076, 1.000000000000000000, 0.9330127018922190762, 0.9330127018922194093 ) ) 
 REPRESENTATION_ITEM ( '' )  );
#2025=CARTESIAN_POINT ( 'NONE',  ( 2.256430356250000546, -2.315624999385482496, 1.302750673588579877 ) ) ;
#2028=VERTEX_POINT ( 'NONE', #79 ) ;
#2034=CARTESIAN_POINT ( 'NONE',  ( 2.256430356250000546, -1.753124999385482496, 1.302750673588579877 ) ) ;
#2035=CARTESIAN_POINT ( 'NONE',  ( -2.500000000000000000, -5.343749998770965348, 0.000000000000000000 ) ) ;
#2036=ORIENTED_EDGE ( 'NONE', *, *, #5758, .F. ) ;
#2038=CARTESIAN_POINT ( 'NONE',  ( -2.256430356250000102, -0.1406249993854829516, 0.000000000000000000 ) ) ;
#2050=CARTESIAN_POINT ( 'NONE',  ( 2.256430356249999658, -0.8906249993854827851, -1.302750673588581432 ) ) ;
#2051=ORIENTED_EDGE ( 'NONE', *, *, #42, .F. ) ;
#2053=CARTESIAN_POINT ( 'NONE',  ( 0.6698729810778075722, -0.7674038105676657118, 2.499999999999999556 ) ) ;
#2054=CARTESIAN_POINT ( 'NONE',  ( 2.500000000000000000, -0.1874999999999999722, -1.443375672974065438 ) ) ;
#2059=CARTESIAN_POINT ( 'NONE',  ( -1.250000000000000222, -0.9187499987709658589, -2.165063509461096825 ) ) ;
#2061=CARTESIAN_POINT ( 'NONE',  ( 2.500000000000000000, -2.924999999999999822, -3.061616997868383141E-16 ) ) ;
#2065=CARTESIAN_POINT ( 'NONE',  ( -0.6698729810778105698, -4.857596189432333844, 2.499999999999997780 ) ) ;
#2068=ORIENTED_EDGE ( 'NONE', *, *, #8907, .F. ) ;
#2069=DIRECTION ( 'NONE',  ( 0.000000000000000000, 0.000000000000000000, -1.000000000000000000 ) ) ;
#2073=CARTESIAN_POINT ( 'NONE',  ( -1.915120254295647362, -5.000523192925935945, -1.606958123781256464 ) ) ;
#2075=ORIENTED_EDGE ( 'NONE', *, *, #5985, .T. ) ;
#2079=CARTESIAN_POINT ( 'NONE',  ( -2.500000000000000000, -2.287499999999999645, -1.443375672974064106 ) ) ;
#2080=AXIS2_PLACEMENT_3D ( 'NONE', #9368, #8475, #2252 ) ;
#2082=PLANE ( 'NONE',  #2080 ) ;
#2083=CARTESIAN_POINT ( 'NONE',  ( 2.256430356249999658, -1.790624999385482807, -1.302750673588581432 ) ) ;
#2086=EDGE_LOOP ( 'NONE', ( #4473, #9500, #7186 ) ) ;
#2093=EDGE_LOOP ( 'NONE', ( #9850, #7032, #5344, #7027, #3006, #9140 ) ) ;
#2094=CARTESIAN_POINT ( 'NONE',  ( 1.128215178125001161, -0.8906249993854828961, 1.954126010382870815 ) ) ;
#2098=( BOUNDED_CURVE ( )  B_SPLINE_CURVE ( 2, ( #1181, #293, #9814, #2650, #1233, #4371, #3485, #4426, #5840 ),
 .UNSPECIFIED., .F., .T. ) 
 B_SPLINE_CURVE_WITH_KNOTS ( ( 3, 2, 2, 2, 3 ),
 ( 0.3125000000000000000, 0.3194444444444444198, 0.3333333333333333148, 0.3472222222222222099, 0.3541666666666666852 ),
 .UNSPECIFIED. ) 
 CURVE ( )  GEOMETRIC_REPRESENTATION_ITEM ( )  RATIONAL_B_SPLINE_CURVE ( ( 0.9330127018922194093, 0.9330127018922194093, 1.000000000000000000, 0.8660254037844387076, 1.000000000000000000, 0.8660254037844387076, 1.000000000000000000, 0.9330127018922190762, 0.9330127018922194093 ) ) 
 REPRESENTATION_ITEM ( '' )  );
#2106=CARTESIAN_POINT ( 'NONE',  ( 4.786228327491941173E-16, -2.840624999385482852, 2.605501347177161087 ) ) ;
#2110=CARTESIAN_POINT ( 'NONE',  ( 9.877377282685029372E-16, -0.3374999999999999667, 2.500000000000000000 ) ) ;
#2112=CARTESIAN_POINT ( 'NONE',  ( 1.128215178125001161, -0.5531249993854828739, 1.954126010382870815 ) ) ;
#2121=ORIENTED_EDGE ( 'NONE', *, *, #1522, .T. ) ;
#2124=CARTESIAN_POINT ( 'NONE',  ( -1.595409442497313560E-16, -0.7031249993854828961, -2.605501347177161087 ) ) ;
#2127=CARTESIAN_POINT ( 'NONE',  ( 0.000000000000000000, -25.00000000000000000, 0.000000000000000000 ) ) ;
#2136=CARTESIAN_POINT ( 'NONE',  ( 2.500000000000000000, -1.125000000000000000, -3.061616997868383141E-16 ) ) ;
#2140=CARTESIAN_POINT ( 'NONE',  ( 2.256430356250000546, -2.765624999385483118, 1.302750673588579877 ) ) ;
#2146=CARTESIAN_POINT ( 'NONE',  ( 2.500000000000000000, -2.024999999999999911, -3.061616997868383141E-16 ) ) ;
#2152=CARTESIAN_POINT ( 'NONE',  ( 2.256430356249999658, -0.7781249993854830738, -1.302750673588581432 ) ) ;
#2154=DIRECTION ( 'NONE',  ( 0.4980973490458726061, -0.08715574274765837404, 0.8627299156628209786 ) ) ;
#2156=ORIENTED_EDGE ( 'NONE', *, *, #3716, .F. ) ;
#2157=CARTESIAN_POINT ( 'NONE',  ( 1.250000000000001110, -2.943749998770965437, 2.165063509461096380 ) ) ;
#2164=ORIENTED_EDGE ( 'NONE', *, *, #6418, .T. ) ;
#2165=CARTESIAN_POINT ( 'NONE',  ( -1.128215178125000273, -0.7781249993854828517, -1.954126010382871259 ) ) ;
#2167=VERTEX_POINT ( 'NONE', #1543 ) ;
#2172=CARTESIAN_POINT ( 'NONE',  ( 2.256430356250000546, -2.315624999385482496, 1.302750673588579877 ) ) ;
#2181=CARTESIAN_POINT ( 'NONE',  ( 0.000000000000000000, -25.00000000000000000, -0.4999999999999968914 ) ) ;
#2182=CARTESIAN_POINT ( 'NONE',  ( 1.128215178125001161, -2.690624999385482941, 1.954126010382870815 ) ) ;
#2183=EDGE_CURVE ( 'NONE', #9074, #2028, #4644, .T. ) ;
#2184=VERTEX_POINT ( 'NONE', #2631 ) ;
#2186=CONICAL_SURFACE ( 'NONE', #6199, 2.500000000000000444, 0.08726646259971666819 ) ;
#2190=ORIENTED_EDGE ( 'NONE', *, *, #2409, .T. ) ;
#2193=CARTESIAN_POINT ( 'NONE',  ( 0.000000000000000000, 0.000000000000000000, 0.000000000000000000 ) ) ;
#2195=CARTESIAN_POINT ( 'NONE',  ( -1.767625397874844694E-16, -3.712499999999999467, -2.886751345948128655 ) ) ;
#2198=CARTESIAN_POINT ( 'NONE',  ( 2.256430356250000102, -0.9281249993854827629, -2.763330213280484622E-16 ) ) ;
#2206=CARTESIAN_POINT ( 'NONE',  ( -1.595409442497313560E-16, -0.2531249993854829961, -2.605501347177161087 ) ) ;
#2212=CARTESIAN_POINT ( 'NONE',  ( -3.486133158594716510E-16, -2.756249998770965437, -2.500000000000000000 ) ) ;
#2220=CARTESIAN_POINT ( 'NONE',  ( 1.128215178124999607, -3.103124999385482585, -1.954126010382871259 ) ) ;
#2221=ORIENTED_EDGE ( 'NONE', *, *, #722, .F. ) ;
#2225=CARTESIAN_POINT ( 'NONE',  ( 1.045839947578414805E-15, -0.5625000000000001110, -2.500000000000000000 ) ) ;
#2227=CARTESIAN_POINT ( 'NONE',  ( 2.256430356250000546, -0.5156249993854828961, 1.302750673588579877 ) ) ;
#2229=VECTOR ( 'NONE', #4667, 1000.000000000000227 ) ;
#2230=CARTESIAN_POINT ( 'NONE',  ( 5.302876193624534821E-16, -2.531249998770965348, 2.886751345948128655 ) ) ;
#2231=VERTEX_POINT ( 'NONE', #8277 ) ;
#2236=CARTESIAN_POINT ( 'NONE',  ( 1.034219503716432668E-14, -4.162500000000000533, -2.500000000000000000 ) ) ;
#2237=CARTESIAN_POINT ( 'NONE',  ( 4.786228327491941173E-16, -2.728124999385482585, 2.605501347177161087 ) ) ;
#2241=CARTESIAN_POINT ( 'NONE',  ( 0.000000000000000000, -25.00000000000000000, 0.000000000000000000 ) ) ;
#2243=DIRECTION ( 'NONE',  ( 0.000000000000000000, 0.000000000000000000, -1.000000000000000000 ) ) ;
#2248=DIRECTION ( 'NONE',  ( 0.000000000000000000, 0.000000000000000000, -1.000000000000000000 ) ) ;
#2250=CARTESIAN_POINT ( 'NONE',  ( -1.915120254295647584, -5.000523192925936833, -1.606958123781256464 ) ) ;
#2252=DIRECTION ( 'NONE',  ( 0.7660496434811018274, 0.000000000000000000, 0.6427814120853811986 ) ) ;
#2253=CARTESIAN_POINT ( 'NONE',  ( -1.128215178125000273, -1.228124999385483029, -1.954126010382871259 ) ) ;
#2263=CARTESIAN_POINT ( 'NONE',  ( 4.786228327491940187E-16, -0.4781249993854829183, 2.605501347177161087 ) ) ;
#2266=CARTESIAN_POINT ( 'NONE',  ( -2.256430356250000102, -2.428124999385482319, -1.302750673588580321 ) ) ;
#2270=APPLICATION_CONTEXT ( 'automotive_design' ) ;
#2273=ORIENTED_EDGE ( 'NONE', *, *, #6979, .T. ) ;
#2274=AXIS2_PLACEMENT_3D ( 'NONE', #2759, #7404, #3382 ) ;
#2278=CARTESIAN_POINT ( 'NONE',  ( -2.256430356249999214, -4.265624999385482674, 1.302750673588581876 ) ) ;
#2279=ORIENTED_EDGE ( 'NONE', *, *, #562, .T. ) ;
#2282=CARTESIAN_POINT ( 'NONE',  ( 2.256430356249999658, -1.340624999385482852, -1.302750673588581432 ) ) ;
#2284=CARTESIAN_POINT ( 'NONE',  ( -0.6698729810778054627, -1.707596189432333933, 2.500000000000000000 ) ) ;
#2285=AXIS2_PLACEMENT_3D ( 'NONE', #660, #5534, #3026 ) ;
#2287=CARTESIAN_POINT ( 'NONE',  ( -1.249999999999998224, -1.218749998770965792, 2.165063509461097713 ) ) ;
#2293=CARTESIAN_POINT ( 'NONE',  ( -1.128215178124998497, -1.865624999385482763, 1.954126010382872147 ) ) ;
#2294=EDGE_CURVE ( 'NONE', #1242, #8813, #2753, .T. ) ;
#2304=CARTESIAN_POINT ( 'NONE',  ( -1.249999999999998224, -3.974999999999999201, 2.165063509461097713 ) ) ;
#2306=CARTESIAN_POINT ( 'NONE',  ( 1.128215178124999607, -4.453124999385482674, -1.954126010382871259 ) ) ;
#2313=CARTESIAN_POINT ( 'NONE',  ( 2.256430356250000102, -3.515624999385482674, -2.763330213280484622E-16 ) ) ;
#2316=CARTESIAN_POINT ( 'NONE',  ( -1.128215178124998497, -2.315624999385482941, 1.954126010382872147 ) ) ;
#2328=CARTESIAN_POINT ( 'NONE',  ( 2.256430356250000546, -4.565624999385482496, 1.302750673588579877 ) ) ;
#2332=CARTESIAN_POINT ( 'NONE',  ( 2.256430356249999658, -2.240624999385482319, -1.302750673588581432 ) ) ;
#2335=PLANE ( 'NONE',  #2285 ) ;
#2336=CARTESIAN_POINT ( 'NONE',  ( 2.500000000000000000, -2.868749998770965703, -3.061616997868383141E-16 ) ) ;
#2340=DIRECTION ( 'NONE',  ( 0.000000000000000000, -1.000000000000000000, 0.000000000000000000 ) ) ;
#2341=CARTESIAN_POINT ( 'NONE',  ( 2.256430356250000546, -1.303124999385482985, 1.302750673588579877 ) ) ;
#2351=CARTESIAN_POINT ( 'NONE',  ( -1.250000000000000222, -3.224999999999999645, -2.165063509461096825 ) ) ;
#2354=CARTESIAN_POINT ( 'NONE',  ( -1.128215178125000273, -3.478124999385482141, -1.954126010382871259 ) ) ;
#2362=CARTESIAN_POINT ( 'NONE',  ( -2.256430356250000102, -4.228124999385483029, -1.302750673588580321 ) ) ;
#2364=EDGE_CURVE ( 'NONE', #4614, #9350, #720, .T. ) ;
#2365=CARTESIAN_POINT ( 'NONE',  ( -2.256430356250000102, -3.328124999385483562, -1.302750673588580321 ) ) ;
#2367=CARTESIAN_POINT ( 'NONE',  ( 3.061616997868383141E-16, 0.000000000000000000, 2.500000000000000000 ) ) ;
#2377=CARTESIAN_POINT ( 'NONE',  ( 2.256430356249999658, -4.940624999385482496, -1.302750673588581432 ) ) ;
#2379=EDGE_CURVE ( 'NONE', #2983, #3142, #2506, .T. ) ;
#2381=CARTESIAN_POINT ( 'NONE',  ( -9.703070624755296135E-15, -4.331249998770966059, 2.500000000000000444 ) ) ;
#2384=CARTESIAN_POINT ( 'NONE',  ( 4.786228327491940187E-16, -3.740624999385481875, 2.605501347177161087 ) ) ;
#2391=CARTESIAN_POINT ( 'NONE',  ( 2.500000000000000444, -1.106249998770965748, 1.443375672974063439 ) ) ;
#2396=CARTESIAN_POINT ( 'NONE',  ( 2.256430356250000546, -4.003124999385482496, 1.302750673588579877 ) ) ;
#2405=CARTESIAN_POINT ( 'NONE',  ( -1.250000000000000222, -3.674999999999999822, -2.165063509461096825 ) ) ;
#2406=CARTESIAN_POINT ( 'NONE',  ( 2.256430356250000546, -4.565624999385482496, 1.302750673588579877 ) ) ;
#2409=EDGE_CURVE ( 'NONE', #2184, #9074, #2098, .T. ) ;
#2414=CARTESIAN_POINT ( 'NONE',  ( -2.256430356250000102, -3.328124999385483562, -1.302750673588580321 ) ) ;
#2416=ORIENTED_EDGE ( 'NONE', *, *, #7857, .F. ) ;
#2417=CARTESIAN_POINT ( 'NONE',  ( 4.786228327491941173E-16, -2.728124999385482585, 2.605501347177161087 ) ) ;
#2420=CARTESIAN_POINT ( 'NONE',  ( -3.486133158594716510E-16, -1.012499999999999956, -2.500000000000000000 ) ) ;
#2427=CARTESIAN_POINT ( 'NONE',  ( -2.256430356249999214, -4.715624999385481964, 1.302750673588581876 ) ) ;
#2428=ORIENTED_EDGE ( 'NONE', *, *, #121, .F. ) ;
#2433=CARTESIAN_POINT ( 'NONE',  ( 2.256430356249999658, -4.940624999385482496, -1.302750673588581432 ) ) ;
#2439=CARTESIAN_POINT ( 'NONE',  ( 2.500000000000000000, -1.518749998770965837, -3.061616997868383141E-16 ) ) ;
#2445=CARTESIAN_POINT ( 'NONE',  ( -1.728525935690056192, -5.141148612710514598, -1.450405475118361043 ) ) ;
#2454=ORIENTED_EDGE ( 'NONE', *, *, #8510, .T. ) ;
#2456=AXIS2_PLACEMENT_3D ( 'NONE', #3728, #9207, #9110 ) ;
#2457=CARTESIAN_POINT ( 'NONE',  ( -3.486133158594716510E-16, -0.5062499987709657701, -2.500000000000000000 ) ) ;
#2458=CARTESIAN_POINT ( 'NONE',  ( 1.128215178124999607, -4.003124999385482496, -1.954126010382871259 ) ) ;
#2465=CARTESIAN_POINT ( 'NONE',  ( -9.703070624755296135E-15, -3.937500000000000888, 2.500000000000000444 ) ) ;
#2468=CARTESIAN_POINT ( 'NONE',  ( 2.256430356250000546, -2.653124999385482852, 1.302750673588579877 ) ) ;
#2472=CARTESIAN_POINT ( 'NONE',  ( -2.500000000000000000, -0.4500000000000000111, 0.000000000000000000 ) ) ;
#2474=LINE ( 'NONE', #6542, #4925 ) ;
#2483=CARTESIAN_POINT ( 'NONE',  ( 2.500000000000000000, -5.081249998770965171, -1.443375672974065438 ) ) ;
#2485=CARTESIAN_POINT ( 'NONE',  ( 1.034219503716432668E-14, -3.656249998770965792, -2.500000000000000000 ) ) ;
#2488=CARTESIAN_POINT ( 'NONE',  ( 1.128215178124999607, -4.003124999385482496, -1.954126010382871259 ) ) ;
#2493=CARTESIAN_POINT ( 'NONE',  ( 2.500000000000000444, -4.706249998770965171, 1.443375672974063439 ) ) ;
#2494=VERTEX_POINT ( 'NONE', #10062 ) ;
#2497=CARTESIAN_POINT ( 'NONE',  ( 3.000000000000000000, -15.00000000000000000, -1.732050807568876749 ) ) ;
#2498=CARTESIAN_POINT ( 'NONE',  ( 2.256430356249999658, -4.828124999385483562, -1.302750673588581432 ) ) ;
#2503=CARTESIAN_POINT ( 'NONE',  ( -1.249999999999998224, -3.524999999999999467, 2.165063509461097713 ) ) ;
#2506=( BOUNDED_CURVE ( )  B_SPLINE_CURVE ( 2, ( #6723, #2065, #5259, #1128, #5152, #10023, #5202 ),
 .UNSPECIFIED., .F., .F. ) 
 B_SPLINE_CURVE_WITH_KNOTS ( ( 3, 2, 2, 3 ),
 ( 0.8958333333333333703, 0.9027777777777777901, 0.9166666666666666297, 0.9258784821878333071 ),
 .UNSPECIFIED. ) 
 CURVE ( )  GEOMETRIC_REPRESENTATION_ITEM ( )  RATIONAL_B_SPLINE_CURVE ( ( 0.9330127018922192983, 0.9330127018922198534, 1.000000000000000000, 0.8660254037844387076, 1.000000000000000000, 0.9111412529300411123, 0.9401537613649495473 ) ) 
 REPRESENTATION_ITEM ( '' )  );
#2508=ORIENTED_EDGE ( 'NONE', *, *, #2556, .F. ) ;
#2512=CARTESIAN_POINT ( 'NONE',  ( -1.128215178124998497, -4.228124999385482141, 1.954126010382872147 ) ) ;
#2513=ORIENTED_EDGE ( 'NONE', *, *, #3854, .F. ) ;
#2521=DIRECTION ( 'NONE',  ( 0.000000000000000000, 0.000000000000000000, -1.000000000000000000 ) ) ;
#2522=CARTESIAN_POINT ( 'NONE',  ( -1.595409442497313560E-16, -4.753124999385482496, -2.605501347177161087 ) ) ;
#2523=CARTESIAN_POINT ( 'NONE',  ( 0.6698729810778050187, -2.567403810567665090, 2.500000000000000444 ) ) ;
#2524=CARTESIAN_POINT ( 'NONE',  ( 4.786228327491941173E-16, -4.528124999385482852, 2.605501347177161087 ) ) ;
#2537=CARTESIAN_POINT ( 'NONE',  ( -2.256430356249998770, -3.365624999385482763, 1.302750673588581876 ) ) ;
#2541=ADVANCED_FACE ( 'NONE', ( #9900 ), #1325, .T. ) ;
#2542=CARTESIAN_POINT ( 'NONE',  ( -1.767625397874844694E-16, -3.656249998770965792, -2.886751345948128655 ) ) ;
#2545=CARTESIAN_POINT ( 'NONE',  ( 0.000000000000000000, -15.00000000000000000, -3.464101615137755275 ) ) ;
#2547=CARTESIAN_POINT ( 'NONE',  ( -2.256430356249999214, -4.603124999385482141, 1.302750673588581876 ) ) ;
#2549=ORIENTED_EDGE ( 'NONE', *, *, #914, .F. ) ;
#2553=DIRECTION ( 'NONE',  ( -0.8660254037844385966, 0.000000000000000000, -0.5000000000000001110 ) ) ;
#2554=CARTESIAN_POINT ( 'NONE',  ( 0.6698729810778112359, -3.676346188203299725, -2.499999999999996447 ) ) ;
#2556=EDGE_CURVE ( 'NONE', #3561, #8603, #7905, .T. ) ;
#2558=CARTESIAN_POINT ( 'NONE',  ( -0.6698729810778054627, -4.407596189432333667, 2.500000000000000000 ) ) ;
#2565=CARTESIAN_POINT ( 'NONE',  ( 4.996790860652426159E-15, -1.462499999999999911, -2.500000000000000000 ) ) ;
#2568=CARTESIAN_POINT ( 'NONE',  ( 2.256430356250000102, -3.965624999385482408, -2.763330213280484622E-16 ) ) ;
#2574=CARTESIAN_POINT ( 'NONE',  ( 0.000000000000000000, 0.000000000000000000, 0.000000000000000000 ) ) ;
#2579=CARTESIAN_POINT ( 'NONE',  ( 0.6698729810778063509, -1.426346188203299947, -2.500000000000000000 ) ) ;
#2581=CARTESIAN_POINT ( 'NONE',  ( 2.256430356250000102, -2.728124999385482585, -2.763330213280484622E-16 ) ) ;
#2583=B_SPLINE_CURVE_WITH_KNOTS ( 'NONE', 1,
 ( #10189, #9510 ),
 .UNSPECIFIED., .F., .F.,
 ( 2, 2 ),
 ( 0.000000000000000000, 1.000000000000000000 ),
 .UNSPECIFIED. ) ;
#2586=CARTESIAN_POINT ( 'NONE',  ( -2.500000000000000000, -5.343749998770965348, 0.000000000000000000 ) ) ;
#2589=CARTESIAN_POINT ( 'NONE',  ( 0.000000000000000000, -25.00000000000000000, 0.000000000000000000 ) ) ;
#2598=LINE ( 'NONE', #4905, #5671 ) ;
#2603=CARTESIAN_POINT ( 'NONE',  ( -1.250000000000000222, -4.574999999999999289, -2.165063509461096825 ) ) ;
#2608=DIRECTION ( 'NONE',  ( -0.4980973490458728836, -0.08715574274765840179, -0.8627299156628209786 ) ) ;
#2612=CARTESIAN_POINT ( 'NONE',  ( 1.250000000000001110, -4.799999999999999822, 2.165063509461096380 ) ) ;
#2613=CARTESIAN_POINT ( 'NONE',  ( -2.500000000000000000, 0.000000000000000000, 0.000000000000000000 ) ) ;
#2614=CARTESIAN_POINT ( 'NONE',  ( 0.000000000000000000, 0.000000000000000000, 0.000000000000000000 ) ) ;
#2617=CARTESIAN_POINT ( 'NONE',  ( 1.250000000000001110, -0.6937499987709658811, 2.165063509461096380 ) ) ;
#2620=CARTESIAN_POINT ( 'NONE',  ( 0.000000000000000000, 0.000000000000000000, -2.500000000000000000 ) ) ;
#2624=EDGE_CURVE ( 'NONE', #9728, #5955, #2881, .T. ) ;
#2631=CARTESIAN_POINT ( 'NONE',  ( 9.877377282685029372E-16, -2.081249998770965615, 2.500000000000000000 ) ) ;
#2634=CARTESIAN_POINT ( 'NONE',  ( -2.499999999999999556, -4.856249998770964638, 1.443375672974065882 ) ) ;
#2640=LINE ( 'NONE', #6661, #10056 ) ;
#2642=CIRCLE ( 'NONE', #8500, 2.062556682370379590 ) ;
#2650=CARTESIAN_POINT ( 'NONE',  ( -2.499999999999999112, -2.156249998770965348, 1.443375672974065882 ) ) ;
#2661=ORIENTED_EDGE ( 'NONE', *, *, #6569, .T. ) ;
#2662=CARTESIAN_POINT ( 'NONE',  ( 1.128215178124999607, -3.440624999385482496, -1.954126010382871259 ) ) ;
#2666=CARTESIAN_POINT ( 'NONE',  ( 0.6698729810778063509, -0.5263461882032999251, -2.500000000000000000 ) ) ;
#2667=DIRECTION ( 'NONE',  ( 0.000000000000000000, 0.000000000000000000, 1.000000000000000000 ) ) ;
#2668=DIRECTION ( 'NONE',  ( 0.000000000000000000, -1.000000000000000000, 0.000000000000000000 ) ) ;
#2670=EDGE_CURVE ( 'NONE', #3656, #1838, #955, .T. ) ;
#2671=ORIENTED_EDGE ( 'NONE', *, *, #1918, .F. ) ;
#2677=CARTESIAN_POINT ( 'NONE',  ( 4.996790860652426159E-15, -1.856249998770965748, -2.500000000000000000 ) ) ;
#2686=CARTESIAN_POINT ( 'NONE',  ( -2.500000000000000000, -3.993749998770965703, 0.000000000000000000 ) ) ;
#2692=CARTESIAN_POINT ( 'NONE',  ( -2.500000000000000000, -0.3937499987709658922, 0.000000000000000000 ) ) ;
#2707=( BOUNDED_SURFACE ( )  B_SPLINE_SURFACE ( 1, 2, ( 
 ( #607, #7718, #1998, #5197, #7775, #3805, #5937, #2745, #3641, #2852, #1951, #9131, #5146, #6037, #2059, #554, #6932, #3131, #7094, #2391, #10351, #3855, #2287, #3908, #3077, #5587, #9607, #7832, #8825, #822, #2439, #3181, #7881, #5634, #7042, #9460, #8773, #4639, #5433, #1654, #8727, #4845, #1551, #8675, #25, #3028, #4741, #713, #6366, #3229, #5536, #8622, #8038, #661, #1600, #10246, #4693, #2230, #871, #4790, #4062, #6319, #1498, #10297, #1446, #9512, #2336, #6261, #7988, #6204, #5485, #769, #10193, #9403, #7936, #3960, #4013, #7147, #9560, #7197, #6417, #9019, #8282, #1012, #8138, #9848, #178, #2542, #9073, #1789, #3324, #8875, #5875, #9658, #4985, #7344, #2686, #1887, #8091, #9750, #7246, #7388, #6513, #1698, #5081, #6606, #135, #4896, #6657, #1113, #83, #3278, #4113, #921, #6467, #2493, #4255, #8923, #5686, #2634, #7298, #3365, #4160, #9798, #228, #9702, #5734, #968, #1742, #5827, #4939, #6560, #2586, #8231, #5778 ),
 ( #8972, #1836, #8184, #4204, #3411, #1062, #5032, #7435, #3470, #276, #329, #4356, #1165, #7710, #2165, #5242, #10121, #2050, #381, #3632, #1219, #4304, #7540, #1941, #3739, #6921, #7490, #2958, #3574, #5136, #3518, #6139, #1326, #5979, #9336, #10063, #5366, #7595, #4411, #6867, #4462, #8335, #6759, #8388, #9957, #2900, #8555, #2791, #6705, #5302, #9902, #7652, #1991, #2737, #489, #433, #5923, #4515, #6812, #3683, #6084, #2844, #8441, #10009, #9275, #9172, #5190, #6029, #545, #2106, #8498, #9121, #9218, #1271, #9391, #3122, #2220, #7871, #8612, #652, #3949, #6194, #6980, #7187, #10288, #6404, #6307, #10234, #1588, #4573, #9503, #9449, #4731, #4780, #7084, #10181, #3218, #5424, #7135, #1437, #6250, #3795, #4003, #10340, #16, #4684, #3066, #2278, #3017, #703, #5474, #4630, #3172, #7768, #7822, #2328, #5624, #9596, #3846, #2427, #6356, #8666, #3896, #599, #9550, #2377, #1381, #5525, #1489, #7031, #8717, #1535, #7925, #757, #5574 ) ),
 .UNSPECIFIED., .F., .F., .F. ) 
 B_SPLINE_SURFACE_WITH_KNOTS ( ( 2, 2 ),
 ( 3, 2, 2, 2, 2, 2, 2, 2, 2, 2, 2, 2, 2, 2, 2, 2, 2, 2, 2, 2, 2, 2, 2, 2, 2, 2, 2, 2, 2, 2, 2, 2, 2, 2, 2, 2, 2, 2, 2, 2, 2, 2, 2, 2, 2, 2, 2, 2, 2, 2, 2, 2, 2, 2, 2, 2, 2, 2, 2, 2, 2, 2, 2, 2, 2, 2, 2, 3 ),
 ( 0.000000000000000000, 1.000000000000000000 ),
 ( 0.000000000000000000, 0.01388888888888888812, 0.02777777777777777624, 0.04166666666666666435, 0.05555555555555555247, 0.06944444444444444753, 0.08333333333333332871, 0.09722222222222222376, 0.1111111111111111049, 0.1250000000000000000, 0.1388888888888888951, 0.1527777777777777901, 0.1666666666666666574, 0.1805555555555555525, 0.1944444444444444475, 0.2083333333333333426, 0.2222222222222222099, 0.2361111111111111049, 0.2500000000000000000, 0.2638888888888888951, 0.2777777777777777901, 0.2916666666666666852, 0.3055555555555555802, 0.3194444444444444198, 0.3333333333333333148, 0.3472222222222222099, 0.3611111111111111049, 0.3750000000000000000, 0.3888888888888888951, 0.4027777777777777901, 0.4166666666666666852, 0.4305555555555555802, 0.4444444444444444198, 0.4583333333333333148, 0.4722222222222222099, 0.4861111111111111049, 0.5000000000000000000, 0.5138888888888888395, 0.5277777777777777901, 0.5416666666666666297, 0.5555555555555555802, 0.5694444444444444198, 0.5833333333333333703, 0.5972222222222222099, 0.6111111111111111605, 0.6250000000000000000, 0.6388888888888888395, 0.6527777777777777901, 0.6666666666666666297, 0.6805555555555555802, 0.6944444444444444198, 0.7083333333333333703, 0.7222222222222222099, 0.7361111111111111605, 0.7500000000000000000, 0.7638888888888888395, 0.7777777777777777901, 0.7916666666666666297, 0.8055555555555555802, 0.8194444444444444198, 0.8333333333333333703, 0.8472222222222222099, 0.8611111111111111605, 0.8750000000000000000, 0.8888888888888888395, 0.9027777777777777901, 0.9166666666666666297, 0.9258784959437954543 ),
 .UNSPECIFIED. ) 
 GEOMETRIC_REPRESENTATION_ITEM ( )  RATIONAL_B_SPLINE_SURFACE ( (
 ( 1.000000000000000000, 0.8660254037844387076, 1.000000000000000000, 0.8660254037844387076, 1.000000000000000000, 0.8660254037844387076, 1.000000000000000000, 0.8660254037844387076, 1.000000000000000000, 0.8660254037844387076, 1.000000000000000000, 0.8660254037844387076, 1.000000000000000000, 0.8660254037844387076, 1.000000000000000000, 0.8660254037844387076, 1.000000000000000000, 0.8660254037844387076, 1.000000000000000000, 0.8660254037844387076, 1.000000000000000000, 0.8660254037844387076, 1.000000000000000000, 0.8660254037844387076, 1.000000000000000000, 0.8660254037844387076, 1.000000000000000000, 0.8660254037844387076, 1.000000000000000000, 0.8660254037844387076, 1.000000000000000000, 0.8660254037844387076, 1.000000000000000000, 0.8660254037844387076, 1.000000000000000000, 0.8660254037844387076, 1.000000000000000000, 0.8660254037844387076, 1.000000000000000000, 0.8660254037844387076, 1.000000000000000000, 0.8660254037844387076, 1.000000000000000000, 0.8660254037844387076, 1.000000000000000000, 0.8660254037844387076, 1.000000000000000000, 0.8660254037844387076, 1.000000000000000000, 0.8660254037844387076, 1.000000000000000000, 0.8660254037844387076, 1.000000000000000000, 0.8660254037844387076, 1.000000000000000000, 0.8660254037844387076, 1.000000000000000000, 0.8660254037844387076, 1.000000000000000000, 0.8660254037844387076, 1.000000000000000000, 0.8660254037844387076, 1.000000000000000000, 0.8660254037844387076, 1.000000000000000000, 0.8660254037844387076, 1.000000000000000000, 0.8660254037844387076, 1.000000000000000000, 0.8660254037844387076, 1.000000000000000000, 0.8660254037844387076, 1.000000000000000000, 0.8660254037844387076, 1.000000000000000000, 0.8660254037844387076, 1.000000000000000000, 0.8660254037844387076, 1.000000000000000000, 0.8660254037844387076, 1.000000000000000000, 0.8660254037844387076, 1.000000000000000000, 0.8660254037844387076, 1.000000000000000000, 0.8660254037844387076, 1.000000000000000000, 0.8660254037844387076, 1.000000000000000000, 0.8660254037844387076, 1.000000000000000000, 0.8660254037844387076, 1.000000000000000000, 0.8660254037844387076, 1.000000000000000000, 0.8660254037844387076, 1.000000000000000000, 0.8660254037844387076, 1.000000000000000000, 0.8660254037844387076, 1.000000000000000000, 0.8660254037844387076, 1.000000000000000000, 0.8660254037844387076, 1.000000000000000000, 0.8660254037844387076, 1.000000000000000000, 0.8660254037844387076, 1.000000000000000000, 0.8660254037844387076, 1.000000000000000000, 0.8660254037844387076, 1.000000000000000000, 0.8660254037844387076, 1.000000000000000000, 0.8660254037844387076, 1.000000000000000000, 0.8660254037844387076, 1.000000000000000000, 0.8660254037844387076, 1.000000000000000000, 0.8660254037844387076, 1.000000000000000000, 0.8660254037844387076, 1.000000000000000000, 0.8660254037844387076, 1.000000000000000000, 0.8660254037844387076, 1.000000000000000000, 0.8660254037844387076, 1.000000000000000000, 0.8660254037844387076, 1.000000000000000000, 0.9111411202376789031, 0.9401538480137057174),
 ( 1.000000000000000000, 0.8660254037844387076, 1.000000000000000000, 0.8660254037844387076, 1.000000000000000000, 0.8660254037844387076, 1.000000000000000000, 0.8660254037844387076, 1.000000000000000000, 0.8660254037844387076, 1.000000000000000000, 0.8660254037844387076, 1.000000000000000000, 0.8660254037844387076, 1.000000000000000000, 0.8660254037844387076, 1.000000000000000000, 0.8660254037844387076, 1.000000000000000000, 0.8660254037844387076, 1.000000000000000000, 0.8660254037844387076, 1.000000000000000000, 0.8660254037844387076, 1.000000000000000000, 0.8660254037844387076, 1.000000000000000000, 0.8660254037844387076, 1.000000000000000000, 0.8660254037844387076, 1.000000000000000000, 0.8660254037844387076, 1.000000000000000000, 0.8660254037844387076, 1.000000000000000000, 0.8660254037844387076, 1.000000000000000000, 0.8660254037844387076, 1.000000000000000000, 0.8660254037844387076, 1.000000000000000000, 0.8660254037844387076, 1.000000000000000000, 0.8660254037844387076, 1.000000000000000000, 0.8660254037844387076, 1.000000000000000000, 0.8660254037844387076, 1.000000000000000000, 0.8660254037844387076, 1.000000000000000000, 0.8660254037844387076, 1.000000000000000000, 0.8660254037844387076, 1.000000000000000000, 0.8660254037844387076, 1.000000000000000000, 0.8660254037844387076, 1.000000000000000000, 0.8660254037844387076, 1.000000000000000000, 0.8660254037844387076, 1.000000000000000000, 0.8660254037844387076, 1.000000000000000000, 0.8660254037844387076, 1.000000000000000000, 0.8660254037844387076, 1.000000000000000000, 0.8660254037844387076, 1.000000000000000000, 0.8660254037844387076, 1.000000000000000000, 0.8660254037844387076, 1.000000000000000000, 0.8660254037844387076, 1.000000000000000000, 0.8660254037844387076, 1.000000000000000000, 0.8660254037844387076, 1.000000000000000000, 0.8660254037844387076, 1.000000000000000000, 0.8660254037844387076, 1.000000000000000000, 0.8660254037844387076, 1.000000000000000000, 0.8660254037844387076, 1.000000000000000000, 0.8660254037844387076, 1.000000000000000000, 0.8660254037844387076, 1.000000000000000000, 0.8660254037844387076, 1.000000000000000000, 0.8660254037844387076, 1.000000000000000000, 0.8660254037844387076, 1.000000000000000000, 0.8660254037844387076, 1.000000000000000000, 0.8660254037844387076, 1.000000000000000000, 0.8660254037844387076, 1.000000000000000000, 0.8660254037844387076, 1.000000000000000000, 0.8660254037844387076, 1.000000000000000000, 0.8660254037844387076, 1.000000000000000000, 0.8660254037844387076, 1.000000000000000000, 0.8660254037844387076, 1.000000000000000000, 0.8660254037844387076, 1.000000000000000000, 0.8660254037844387076, 1.000000000000000000, 0.8660254037844387076, 1.000000000000000000, 0.8660254037844387076, 1.000000000000000000, 0.8660254037844387076, 1.000000000000000000, 0.8660254037844387076, 1.000000000000000000, 0.8660254037844387076, 1.000000000000000000, 0.8660254037844387076, 1.000000000000000000, 0.8660254037844387076, 1.000000000000000000, 0.9111411202376789031, 0.9401538480137057174) ) ) 
 REPRESENTATION_ITEM ( '' )  SURFACE ( )  );
#2708=CARTESIAN_POINT ( 'NONE',  ( 3.061616997868383141E-16, 0.000000000000000000, 2.500000000000000000 ) ) ;
#2710=CARTESIAN_POINT ( 'NONE',  ( 9.877377282685029372E-16, -0.3374999999999999667, 2.500000000000000000 ) ) ;
#2713=CARTESIAN_POINT ( 'NONE',  ( -2.256430356249998770, -5.053124999385482319, 1.302750673588581876 ) ) ;
#2715=CARTESIAN_POINT ( 'NONE',  ( -2.499999999999999556, -0.8624999999999998224, 1.443375672974065882 ) ) ;
#2716=CARTESIAN_POINT ( 'NONE',  ( -2.500000000000000000, -2.699999999999999734, 0.000000000000000000 ) ) ;
#2717=CARTESIAN_POINT ( 'NONE',  ( -1.128215178125000273, -0.3281249993854828961, -1.954126010382871259 ) ) ;
#2719=CARTESIAN_POINT ( 'NONE',  ( -2.500000000000000000, -0.9000000000000000222, 0.000000000000000000 ) ) ;
#2721=LINE ( 'NONE', #1925, #6603 ) ;
#2732=ADVANCED_FACE ( 'NONE', ( #2832 ), #3671, .T. ) ;
#2735=ORIENTED_EDGE ( 'NONE', *, *, #5617, .F. ) ;
#2737=CARTESIAN_POINT ( 'NONE',  ( 2.256430356249999658, -2.240624999385482319, -1.302750673588581432 ) ) ;
#2740=CARTESIAN_POINT ( 'NONE',  ( -4.357666448243394824E-15, -2.587499999999999467, 2.500000000000000000 ) ) ;
#2745=CARTESIAN_POINT ( 'NONE',  ( 2.500000000000000444, -0.6562499987709659033, 1.443375672974063439 ) ) ;
#2753=LINE ( 'NONE', #397, #4061 ) ;
#2756=LINE ( 'NONE', #197, #2947 ) ;
#2759=CARTESIAN_POINT ( 'NONE',  ( 0.000000000000000000, -20.00000000000000000, 0.000000000000000000 ) ) ;
#2762=DIRECTION ( 'NONE',  ( 0.000000000000000000, 0.000000000000000000, -1.000000000000000000 ) ) ;
#2764=CARTESIAN_POINT ( 'NONE',  ( -2.500000000000000000, -0.4500000000000000111, 0.000000000000000000 ) ) ;
#2768=CARTESIAN_POINT ( 'NONE',  ( -1.250000000000000222, -0.9749999999999999778, -2.165063509461096825 ) ) ;
#2770=DIRECTION ( 'NONE',  ( 0.000000000000000000, 0.000000000000000000, -1.000000000000000000 ) ) ;
#2774=CARTESIAN_POINT ( 'NONE',  ( 9.877377282685029372E-16, -0.7312499987709657479, 2.500000000000000000 ) ) ;
#2775=ORIENTED_EDGE ( 'NONE', *, *, #8873, .F. ) ;
#2781=CARTESIAN_POINT ( 'NONE',  ( 3.000000000000000000, -15.00000000000000000, 1.732050807568879192 ) ) ;
#2787=ORIENTED_EDGE ( 'NONE', *, *, #1705, .F. ) ;
#2791=CARTESIAN_POINT ( 'NONE',  ( -2.256430356249999214, -2.015624999385482674, 1.302750673588581876 ) ) ;
#2800=ORIENTED_EDGE ( 'NONE', *, *, #6106, .T. ) ;
#2802=CARTESIAN_POINT ( 'NONE',  ( -3.486133158594716510E-16, -2.756249998770965437, -2.500000000000000000 ) ) ;
#2803=CARTESIAN_POINT ( 'NONE',  ( 1.249999999999999334, -2.399999999999999911, -2.165063509461096825 ) ) ;
#2806=MANIFOLD_SOLID_BREP ( 'Thread1', #1623 ) ;
#2813=FACE_BOUND ( 'NONE', #1488, .T. ) ;
#2824=CARTESIAN_POINT ( 'NONE',  ( 2.500000000000000000, -1.987499999999999600, -1.443375672974064994 ) ) ;
#2826=CARTESIAN_POINT ( 'NONE',  ( -3.486133158594716510E-16, -3.712499999999999467, -2.500000000000000000 ) ) ;
#2827=CARTESIAN_POINT ( 'NONE',  ( 1.128215178125001161, -2.353124999385482585, 1.954126010382870815 ) ) ;
#2830=VERTEX_POINT ( 'NONE', #5460 ) ;
#2832=FACE_OUTER_BOUND ( 'NONE', #1997, .T. ) ;
#2833=FACE_OUTER_BOUND ( 'NONE', #1989, .T. ) ;
#2834=CARTESIAN_POINT ( 'NONE',  ( -1.595409442497313560E-16, -2.503124999385482496, -2.605501347177161087 ) ) ;
#2835=CARTESIAN_POINT ( 'NONE',  ( -0.6698729810778105698, -3.957596189432334377, 2.499999999999997780 ) ) ;
#2837=( BOUNDED_CURVE ( )  B_SPLINE_CURVE ( 2, ( #2826, #4547, #524, #6170, #3044, #5340, #5218, #4659, #7627 ),
 .UNSPECIFIED., .F., .T. ) 
 B_SPLINE_CURVE_WITH_KNOTS ( ( 3, 2, 2, 2, 3 ),
 ( 0.6875000000000000000, 0.6944444444444444198, 0.7083333333333333703, 0.7222222222222222099, 0.7291666666666667407 ),
 .UNSPECIFIED. ) 
 CURVE ( )  GEOMETRIC_REPRESENTATION_ITEM ( )  RATIONAL_B_SPLINE_CURVE ( ( 0.9330127018922194093, 0.9330127018922194093, 1.000000000000000000, 0.8660254037844387076, 1.000000000000000000, 0.8660254037844387076, 1.000000000000000000, 0.9330127018922187432, 0.9330127018922192983 ) ) 
 REPRESENTATION_ITEM ( '' )  );
#2839=CARTESIAN_POINT ( 'NONE',  ( -1.249999999999998224, -1.668749998770965970, 2.165063509461097713 ) ) ;
#2844=CARTESIAN_POINT ( 'NONE',  ( -2.256430356250000102, -2.540624999385482141, -1.302750673588580321 ) ) ;
#2847=LINE ( 'NONE', #9221, #9794 ) ;
#2852=CARTESIAN_POINT ( 'NONE',  ( 5.302876193624534821E-16, -0.7312499987709658589, 2.886751345948128655 ) ) ;
#2853=CARTESIAN_POINT ( 'NONE',  ( -2.500000000000000000, -2.681249998770965259, -1.443375672974064106 ) ) ;
#2856=CARTESIAN_POINT ( 'NONE',  ( -1.002171269888535572E-15, -20.00000000000000000, 2.958985580760426615 ) ) ;
#2860=EDGE_CURVE ( 'NONE', #3761, #7541, #10218, .T. ) ;
#2862=ORIENTED_EDGE ( 'NONE', *, *, #6832, .F. ) ;
#2867=CARTESIAN_POINT ( 'NONE',  ( -1.250000000000000222, -0.5250000000000000222, -2.165063509461096825 ) ) ;
#2873=CARTESIAN_POINT ( 'NONE',  ( -1.250000000000000222, -1.875000000000000000, -2.165063509461096825 ) ) ;
#2875=CARTESIAN_POINT ( 'NONE',  ( -1.595409442497313560E-16, -2.165624999385483029, -2.605501347177161087 ) ) ;
#2881=CIRCLE ( 'NONE', #8073, 2.500000000000000000 ) ;
#2883=CARTESIAN_POINT ( 'NONE',  ( -1.249999999999998224, -3.018749998770965615, 2.165063509461097713 ) ) ;
#2886=CARTESIAN_POINT ( 'NONE',  ( -1.128215178124998497, -2.315624999385482941, 1.954126010382872147 ) ) ;
#2891=AXIS2_PLACEMENT_3D ( 'NONE', #3504, #8322, #6690 ) ;
#2900=CARTESIAN_POINT ( 'NONE',  ( 4.786228327491941173E-16, -1.940624999385482718, 2.605501347177161087 ) ) ;
#2905=CARTESIAN_POINT ( 'NONE',  ( 2.256430356250000546, -0.9656249993854827407, 1.302750673588579877 ) ) ;
#2915=CARTESIAN_POINT ( 'NONE',  ( -2.256430356249999214, -1.453124999385482896, 1.302750673588581876 ) ) ;
#2921=CARTESIAN_POINT ( 'NONE',  ( 0.000000000000000000, 0.000000000000000000, -2.500000000000000000 ) ) ;
#2926=VERTEX_POINT ( 'NONE', #2465 ) ;
#2928=CARTESIAN_POINT ( 'NONE',  ( 2.500000000000000000, -1.537499999999999645, -1.443375672974064994 ) ) ;
#2933=CARTESIAN_POINT ( 'NONE',  ( 4.786228327491941173E-16, -2.840624999385482852, 2.605501347177161087 ) ) ;
#2936=ORIENTED_EDGE ( 'NONE', *, *, #2624, .T. ) ;
#2943=CARTESIAN_POINT ( 'NONE',  ( -1.595409442497313560E-16, -2.053124999385482763, -2.605501347177161087 ) ) ;
#2947=VECTOR ( 'NONE', #5750, 1000.000000000000000 ) ;
#2950=ORIENTED_EDGE ( 'NONE', *, *, #9357, .F. ) ;
#2951=CARTESIAN_POINT ( 'NONE',  ( 2.500000000000000000, -2.868749998770965703, -3.061616997868383141E-16 ) ) ;
#2953=CARTESIAN_POINT ( 'NONE',  ( -9.703070624755296135E-15, -3.881249998770965881, 2.500000000000000444 ) ) ;
#2954=VERTEX_POINT ( 'NONE', #2565 ) ;
#2958=CARTESIAN_POINT ( 'NONE',  ( -1.595409442497313560E-16, -1.265624999385482896, -2.605501347177161087 ) ) ;
#2966=CARTESIAN_POINT ( 'NONE',  ( 2.256430356249999658, -0.8906249993854827851, -1.302750673588581432 ) ) ;
#2968=CARTESIAN_POINT ( 'NONE',  ( -1.249999999999998224, -1.724999999999999645, 2.165063509461097713 ) ) ;
#2973=ORIENTED_EDGE ( 'NONE', *, *, #4900, .T. ) ;
#2975=DIRECTION ( 'NONE',  ( 0.000000000000000000, -1.000000000000000000, 0.000000000000000000 ) ) ;
#2976=CARTESIAN_POINT ( 'NONE',  ( 1.128215178124999607, -1.190624999385482941, -1.954126010382871259 ) ) ;
#2983=VERTEX_POINT ( 'NONE', #6489 ) ;
#2988=CARTESIAN_POINT ( 'NONE',  ( 5.302876193624534821E-16, -3.037499999999999645, 2.886751345948128655 ) ) ;
#2991=CARTESIAN_POINT ( 'NONE',  ( 2.256430356249999658, -2.690624999385482941, -1.302750673588581432 ) ) ;
#2997=EDGE_CURVE ( 'NONE', #3336, #1808, #4959, .T. ) ;
#3004=CARTESIAN_POINT ( 'NONE',  ( 2.256430356250000546, -1.303124999385482985, 1.302750673588579877 ) ) ;
#3006=ORIENTED_EDGE ( 'NONE', *, *, #1918, .T. ) ;
#3007=CARTESIAN_POINT ( 'NONE',  ( 1.128215178124999607, -0.2906249993854829738, -1.954126010382871259 ) ) ;
#3013=ORIENTED_EDGE ( 'NONE', *, *, #2379, .F. ) ;
#3017=CARTESIAN_POINT ( 'NONE',  ( -2.256430356250000102, -4.303124999385482319, 0.000000000000000000 ) ) ;
#3020=CARTESIAN_POINT ( 'NONE',  ( 9.877377282685029372E-16, -0.7874999999999998668, 2.500000000000000000 ) ) ;
#3022=PRODUCT ( 'grease nipple', 'grease nipple', '', ( #572 ) ) ;
#3024=CARTESIAN_POINT ( 'NONE',  ( -2.256430356250000102, -1.603124999385482807, 0.000000000000000000 ) ) ;
#3026=DIRECTION ( 'NONE',  ( 0.000000000000000000, -0.000000000000000000, -1.000000000000000000 ) ) ;
#3028=CARTESIAN_POINT ( 'NONE',  ( 5.302876193624534821E-16, -2.081249998770965171, 2.886751345948128655 ) ) ;
#3029=ADVANCED_FACE ( 'NONE', ( #4871 ), #8060, .T. ) ;
#3034=CARTESIAN_POINT ( 'NONE',  ( -2.256430356250000102, -1.940624999385482941, 0.000000000000000000 ) ) ;
#3037=CARTESIAN_POINT ( 'NONE',  ( -1.915120254295647362, -5.000523192925935945, -1.606958123781256464 ) ) ;
#3043=CARTESIAN_POINT ( 'NONE',  ( 1.249999999999999334, -4.200000000000000178, -2.165063509461096825 ) ) ;
#3044=CARTESIAN_POINT ( 'NONE',  ( 2.500000000000000000, -3.824999999999999734, -3.061616997868383141E-16 ) ) ;
#3045=CARTESIAN_POINT ( 'NONE',  ( -1.128215178125000273, -0.7781249993854828517, -1.954126010382871259 ) ) ;
#3049=CARTESIAN_POINT ( 'NONE',  ( -2.499999999999999112, -3.056249998770965703, 1.443375672974065882 ) ) ;
#3051=DIRECTION ( 'NONE',  ( 0.000000000000000000, -1.000000000000000000, 0.000000000000000000 ) ) ;
#3052=CARTESIAN_POINT ( 'NONE',  ( -1.128215178124998497, -0.9656249993854828517, 1.954126010382872147 ) ) ;
#3053=LINE ( 'NONE', #9584, #4947 ) ;
#3056=CARTESIAN_POINT ( 'NONE',  ( -1.595409442497313560E-16, -1.603124999385482807, -2.605501347177161087 ) ) ;
#3066=CARTESIAN_POINT ( 'NONE',  ( -1.128215178124998497, -4.228124999385482141, 1.954126010382872147 ) ) ;
#3072=EDGE_CURVE ( 'NONE', #7399, #9350, #8305, .T. ) ;
#3073=CARTESIAN_POINT ( 'NONE',  ( -2.256430356249998770, -1.115624999385482763, 1.302750673588581876 ) ) ;
#3074=DIRECTION ( 'NONE',  ( -0.000000000000000000, -0.000000000000000000, -1.000000000000000000 ) ) ;
#3076=AXIS2_PLACEMENT_3D ( 'NONE', #9135, #3483, #3698 ) ;
#3077=CARTESIAN_POINT ( 'NONE',  ( -2.500000000000000000, -1.293749998770965970, 0.000000000000000000 ) ) ;
#3078=ORIENTED_EDGE ( 'NONE', *, *, #4198, .T. ) ;
#3084=CARTESIAN_POINT ( 'NONE',  ( 4.786228327491941173E-16, -1.828124999385482896, 2.605501347177161087 ) ) ;
#3085=ORIENTED_EDGE ( 'NONE', *, *, #4556, .T. ) ;
#3089=CARTESIAN_POINT ( 'NONE',  ( 0.000000000000000000, -15.00000000000000000, -3.464101615137755275 ) ) ;
#3096=ADVANCED_FACE ( 'NONE', ( #5954 ), #9146, .T. ) ;
#3097=CARTESIAN_POINT ( 'NONE',  ( -2.500000000000000000, -3.149999999999999467, 0.000000000000000000 ) ) ;
#3099=CARTESIAN_POINT ( 'NONE',  ( -2.256430356250000102, -4.790624999385483029, -1.302750673588580321 ) ) ;
#3108=CARTESIAN_POINT ( 'NONE',  ( 3.000000000000000000, -15.00000000000000000, -1.732050807568876749 ) ) ;
#3109=CARTESIAN_POINT ( 'NONE',  ( 2.256430356250000102, -4.865624999385482319, -2.763330213280484622E-16 ) ) ;
#3111=VERTEX_POINT ( 'NONE', #3600 ) ;
#3113=CARTESIAN_POINT ( 'NONE',  ( 2.256430356249999658, -2.128124999385482941, -1.302750673588581432 ) ) ;
#3122=CARTESIAN_POINT ( 'NONE',  ( -1.595409442497313560E-16, -3.065624999385482496, -2.605501347177161087 ) ) ;
#3125=CARTESIAN_POINT ( 'NONE',  ( 3.061616997868383141E-16, 0.000000000000000000, 2.500000000000000000 ) ) ;
#3126=CARTESIAN_POINT ( 'NONE',  ( -2.256430356250000102, -1.153124999385482852, 0.000000000000000000 ) ) ;
#3128=ORIENTED_EDGE ( 'NONE', *, *, #103, .F. ) ;
#3131=CARTESIAN_POINT ( 'NONE',  ( 2.500000000000000000, -1.031249998770965792, -1.443375672974064994 ) ) ;
#3135=CARTESIAN_POINT ( 'NONE',  ( 1.250000000000001110, -4.349999999999999645, 2.165063509461096380 ) ) ;
#3136=CARTESIAN_POINT ( 'NONE',  ( -1.595409442497313560E-16, -2.503124999385482496, -2.605501347177161087 ) ) ;
#3139=AXIS2_PLACEMENT_3D ( 'NONE', #6934, #1228, #555 ) ;
#3140=EDGE_CURVE ( 'NONE', #9216, #6035, #8863, .T. ) ;
#3142=VERTEX_POINT ( 'NONE', #2073 ) ;
#3147=CARTESIAN_POINT ( 'NONE',  ( -2.499999999999999556, -4.462499999999999467, 1.443375672974065882 ) ) ;
#3152=CARTESIAN_POINT ( 'NONE',  ( 2.256430356250000102, -4.078124999385482674, -2.763330213280484622E-16 ) ) ;
#3153=EDGE_CURVE ( 'NONE', #2830, #5524, #5268, .T. ) ;
#3160=CARTESIAN_POINT ( 'NONE',  ( 1.128215178125001161, -3.140624999385482674, 1.954126010382870815 ) ) ;
#3162=CARTESIAN_POINT ( 'NONE',  ( -1.128215178124998497, -3.215624999385482408, 1.954126010382872147 ) ) ;
#3171=VERTEX_POINT ( 'NONE', #494 ) ;
#3172=CARTESIAN_POINT ( 'NONE',  ( 1.128215178124999607, -4.453124999385482674, -1.954126010382871259 ) ) ;
#3177=CARTESIAN_POINT ( 'NONE',  ( -1.128215178124998497, -3.778124999385482408, 1.954126010382872147 ) ) ;
#3181=CARTESIAN_POINT ( 'NONE',  ( 2.500000000000000444, -1.556249998770965925, 1.443375672974063439 ) ) ;
#3184=CARTESIAN_POINT ( 'NONE',  ( -2.500000000000000000, -4.481249998770965526, -1.443375672974064106 ) ) ;
#3185=( BOUNDED_CURVE ( )  B_SPLINE_CURVE ( 2, ( #1275, #4633, #6088, #2054, #7036, #1385, #7826, #602, #2110 ),
 .UNSPECIFIED., .F., .T. ) 
 B_SPLINE_CURVE_WITH_KNOTS ( ( 3, 2, 2, 2, 3 ),
 ( 0.02083333333333333565, 0.02777777777777777624, 0.04166666666666666435, 0.05555555555555555247, 0.06250000000000000000 ),
 .UNSPECIFIED. ) 
 CURVE ( )  GEOMETRIC_REPRESENTATION_ITEM ( )  RATIONAL_B_SPLINE_CURVE ( ( 0.9330127018922194093, 0.9330127018922194093, 1.000000000000000000, 0.8660254037844387076, 1.000000000000000000, 0.8660254037844387076, 1.000000000000000000, 0.9330127018922194093, 0.9330127018922194093 ) ) 
 REPRESENTATION_ITEM ( '' )  );
#3186=CARTESIAN_POINT ( 'NONE',  ( -2.256430356250000102, -2.878124999385482941, -1.302750673588580321 ) ) ;
#3189=EDGE_LOOP ( 'NONE', ( #1395, #3381, #4742, #5806, #2051, #5447, #9134, #947, #3412, #991, #3971, #7508, #1405, #3575, #7924, #5695, #5542, #290, #1220, #31, #692, #9551, #7080, #6301, #9958, #4852 ) ) ;
#3192=CARTESIAN_POINT ( 'NONE',  ( 1.249999999999999334, -1.893749998770965837, -2.165063509461096825 ) ) ;
#3196=CARTESIAN_POINT ( 'NONE',  ( -1.767625397874844694E-16, -4.162499999999999645, -2.886751345948128655 ) ) ;
#3199=CARTESIAN_POINT ( 'NONE',  ( 2.256430356249999658, -3.590624999385481964, -1.302750673588581432 ) ) ;
#3205=PLANE ( 'NONE',  #5965 ) ;
#3206=CARTESIAN_POINT ( 'NONE',  ( -1.595409442497313560E-16, -4.303124999385482319, -2.605501347177161087 ) ) ;
#3210=CARTESIAN_POINT ( 'NONE',  ( -2.256430356249999214, -2.803124999385482763, 1.302750673588581876 ) ) ;
#3218=CARTESIAN_POINT ( 'NONE',  ( -2.256430356250000102, -3.853124999385482585, 0.000000000000000000 ) ) ;
#3224=CARTESIAN_POINT ( 'NONE',  ( 2.256430356249999658, -4.040624999385483029, -1.302750673588581432 ) ) ;
#3229=CARTESIAN_POINT ( 'NONE',  ( -2.500000000000000000, -2.231249998770965970, -1.443375672974064106 ) ) ;
#3231=CARTESIAN_POINT ( 'NONE',  ( 1.250000000000001110, -1.143749998770965837, 2.165063509461096380 ) ) ;
#3234=CARTESIAN_POINT ( 'NONE',  ( 4.786228327491941173E-16, -4.978124999385483029, 2.605501347177161087 ) ) ;
#3246=CARTESIAN_POINT ( 'NONE',  ( -1.128215178125000273, -4.378124999385482496, -1.954126010382871259 ) ) ;
#3249=CARTESIAN_POINT ( 'NONE',  ( -3.486133158594716510E-16, -1.406249998770965570, -2.500000000000000000 ) ) ;
#3254=CARTESIAN_POINT ( 'NONE',  ( -2.256430356250000102, -4.640624999385482674, 0.000000000000000000 ) ) ;
#3257=ORIENTED_EDGE ( 'NONE', *, *, #7088, .F. ) ;
#3258=CARTESIAN_POINT ( 'NONE',  ( 1.128215178124999607, -1.640624999385482896, -1.954126010382871259 ) ) ;
#3262=CARTESIAN_POINT ( 'NONE',  ( 2.500000000000000000, -3.318749998770965437, -3.061616997868383141E-16 ) ) ;
#3264=EDGE_CURVE ( 'NONE', #1900, #9216, #3185, .T. ) ;
#3270=LINE ( 'NONE', #6462, #7245 ) ;
#3271=CARTESIAN_POINT ( 'NONE',  ( -2.256430356250000102, -4.790624999385483918, -1.302750673588580321 ) ) ;
#3276=EDGE_CURVE ( 'NONE', #1380, #3621, #3799, .T. ) ;
#3277=EDGE_CURVE ( 'NONE', #4882, #1444, #234, .T. ) ;
#3278=CARTESIAN_POINT ( 'NONE',  ( -1.767625397874844694E-16, -4.556249998770965703, -2.886751345948128655 ) ) ;
#3281=CARTESIAN_POINT ( 'NONE',  ( 0.6698729810778069060, -0.9763461882033002137, -2.500000000000000000 ) ) ;
#3284=CARTESIAN_POINT ( 'NONE',  ( -2.256430356250000102, -2.840624999385482852, 0.000000000000000000 ) ) ;
#3286=VERTEX_POINT ( 'NONE', #7087 ) ;
#3287=CARTESIAN_POINT ( 'NONE',  ( 0.6698729810778075722, -1.667403810567665623, 2.499999999999999556 ) ) ;
#3293=CARTESIAN_POINT ( 'NONE',  ( 2.256430356250000102, -3.628124999385482496, -2.763330213280484622E-16 ) ) ;
#3302=CARTESIAN_POINT ( 'NONE',  ( -1.595409442497313560E-16, -2.953124999385483118, -2.605501347177161087 ) ) ;
#3305=CARTESIAN_POINT ( 'NONE',  ( -2.256430356250000102, -3.740624999385482763, 0.000000000000000000 ) ) ;
#3308=LINE ( 'NONE', #2367, #10118 ) ;
#3319=CARTESIAN_POINT ( 'NONE',  ( 2.256430356250000546, -3.215624999385482408, 1.302750673588579877 ) ) ;
#3321=EDGE_CURVE ( 'NONE', #1380, #9254, #641, .T. ) ;
#3323=CARTESIAN_POINT ( 'NONE',  ( 1.034219503716432668E-14, -4.612500000000000711, -2.500000000000000000 ) ) ;
#3324=CARTESIAN_POINT ( 'NONE',  ( 2.500000000000000000, -3.768749998770965171, -3.061616997868383141E-16 ) ) ;
#3325=ORIENTED_EDGE ( 'NONE', *, *, #2860, .F. ) ;
#3328=( BOUNDED_CURVE ( )  B_SPLINE_CURVE ( 2, ( #1663, #4857, #2503, #3528, #6615, #1122, #3422, #1751, #4994 ),
 .UNSPECIFIED., .F., .F. ) 
 B_SPLINE_CURVE_WITH_KNOTS ( ( 3, 2, 2, 2, 3 ),
 ( 0.6458333333333333703, 0.6527777777777777901, 0.6666666666666666297, 0.6805555555555555802, 0.6875000000000000000 ),
 .UNSPECIFIED. ) 
 CURVE ( )  GEOMETRIC_REPRESENTATION_ITEM ( )  RATIONAL_B_SPLINE_CURVE ( ( 0.9330127018922192983, 0.9330127018922198534, 1.000000000000000000, 0.8660254037844387076, 1.000000000000000000, 0.8660254037844387076, 1.000000000000000000, 0.9330127018922194093, 0.9330127018922194093 ) ) 
 REPRESENTATION_ITEM ( '' )  );
#3331=CARTESIAN_POINT ( 'NONE',  ( -1.595409442497313560E-16, -3.853124999385482585, -2.605501347177161087 ) ) ;
#3336=VERTEX_POINT ( 'NONE', #2485 ) ;
#3338=CARTESIAN_POINT ( 'NONE',  ( -2.499999999999999112, -4.462499999999999467, 1.443375672974065882 ) ) ;
#3343=CARTESIAN_POINT ( 'NONE',  ( 2.500000000000000000, -4.668749998770964638, -3.061616997868383141E-16 ) ) ;
#3346=CARTESIAN_POINT ( 'NONE',  ( 9.877377282685029372E-16, -4.781249998770965348, 2.500000000000000000 ) ) ;
#3349=CARTESIAN_POINT ( 'NONE',  ( -1.595409442497313560E-16, -4.303124999385482319, -2.605501347177161087 ) ) ;
#3350=FILL_AREA_STYLE ('',( #5808 ) ) ;
#3351=CARTESIAN_POINT ( 'NONE',  ( 0.000000000000000000, 0.000000000000000000, 0.000000000000000000 ) ) ;
#3353=CARTESIAN_POINT ( 'NONE',  ( 0.6698729810778075722, -3.411153809338631326, 2.499999999999999556 ) ) ;
#3354=CARTESIAN_POINT ( 'NONE',  ( -2.499999999999999112, -1.312499999999999778, 1.443375672974065882 ) ) ;
#3355=CARTESIAN_POINT ( 'NONE',  ( -9.703070624755296135E-15, -3.487499999999999822, 2.500000000000000444 ) ) ;
#3359=LINE ( 'NONE', #7288, #10143 ) ;
#3361=CARTESIAN_POINT ( 'NONE',  ( 2.256430356250000546, -4.115624999385482319, 1.302750673588579877 ) ) ;
#3365=CARTESIAN_POINT ( 'NONE',  ( -2.500000000000000000, -4.931249998770966592, -1.443375672974064106 ) ) ;
#3368=FACE_OUTER_BOUND ( 'NONE', #5665, .T. ) ;
#3371=CARTESIAN_POINT ( 'NONE',  ( -2.256430356250000102, -3.328124999385483562, -1.302750673588580321 ) ) ;
#3372=VERTEX_POINT ( 'NONE', #5972 ) ;
#3381=ORIENTED_EDGE ( 'NONE', *, *, #3951, .T. ) ;
#3382=DIRECTION ( 'NONE',  ( 0.000000000000000000, -0.000000000000000000, -1.000000000000000000 ) ) ;
#3394=CARTESIAN_POINT ( 'NONE',  ( -1.128215178125000273, -4.265624999385482674, -1.954126010382871259 ) ) ;
#3411=CARTESIAN_POINT ( 'NONE',  ( 1.128215178124999607, -0.4031249993854829627, -1.954126010382871259 ) ) ;
#3412=ORIENTED_EDGE ( 'NONE', *, *, #3321, .F. ) ;
#3422=CARTESIAN_POINT ( 'NONE',  ( -1.250000000000000222, -3.674999999999999822, -2.165063509461096825 ) ) ;
#3423=DIRECTION ( 'NONE',  ( -0.9961946980917455452, -0.08715574274765837404, 0.000000000000000000 ) ) ;
#3434=( BOUNDED_CURVE ( )  B_SPLINE_CURVE ( 2, ( #7520, #3446, #5809, #311, #2716, #7369, #1971, #9000, #6635 ),
 .UNSPECIFIED., .F., .F. ) 
 B_SPLINE_CURVE_WITH_KNOTS ( ( 3, 2, 2, 2, 3 ),
 ( 0.4791666666666666852, 0.4861111111111111049, 0.5000000000000000000, 0.5138888888888888395, 0.5208333333333333703 ),
 .UNSPECIFIED. ) 
 CURVE ( )  GEOMETRIC_REPRESENTATION_ITEM ( )  RATIONAL_B_SPLINE_CURVE ( ( 0.9330127018922194093, 0.9330127018922196314, 1.000000000000000000, 0.8660254037844387076, 1.000000000000000000, 0.8660254037844387076, 1.000000000000000000, 0.9330127018922187432, 0.9330127018922192983 ) ) 
 REPRESENTATION_ITEM ( '' )  );
#3440=CARTESIAN_POINT ( 'NONE',  ( 2.500000000000000000, -4.687500000000000000, -1.443375672974065438 ) ) ;
#3441=CIRCLE ( 'NONE', #4449, 2.500000000000000000 ) ;
#3443=CARTESIAN_POINT ( 'NONE',  ( -1.767625397874844694E-16, -0.1124999999999999889, -2.886751345948128655 ) ) ;
#3444=ADVANCED_FACE ( 'NONE', ( #5915 ), #7428, .T. ) ;
#3446=CARTESIAN_POINT ( 'NONE',  ( -0.6698729810778081273, -2.607596189432333844, 2.499999999999999112 ) ) ;
#3449=ADVANCED_FACE ( 'NONE', ( #5180 ), #8733, .T. ) ;
#3460=CARTESIAN_POINT ( 'NONE',  ( 0.000000000000000000, -20.00000000000000000, 0.000000000000000000 ) ) ;
#3462=CARTESIAN_POINT ( 'NONE',  ( -1.250000000000000222, -1.818749998770965881, -2.165063509461096825 ) ) ;
#3465=EDGE_CURVE ( 'NONE', #3621, #2231, #1022, .T. ) ;
#3470=CARTESIAN_POINT ( 'NONE',  ( 1.128215178125001161, -0.5531249993854828739, 1.954126010382870815 ) ) ;
#3471=ORIENTED_EDGE ( 'NONE', *, *, #9811, .T. ) ;
#3472=AXIS2_PLACEMENT_3D ( 'NONE', #4049, #6401, #8078 ) ;
#3473=LINE ( 'NONE', #1745, #6303 ) ;
#3479=ADVANCED_FACE ( 'NONE', ( #774 ), #1341, .T. ) ;
#3483=DIRECTION ( 'NONE',  ( 0.000000000000000000, -1.000000000000000000, 0.000000000000000000 ) ) ;
#3485=CARTESIAN_POINT ( 'NONE',  ( -1.250000000000000222, -2.268749998770965615, -2.165063509461096825 ) ) ;
#3497=CARTESIAN_POINT ( 'NONE',  ( -1.249999999999998224, -0.3749999999999999445, 2.165063509461097713 ) ) ;
#3504=CARTESIAN_POINT ( 'NONE',  ( 0.000000000000000000, 0.000000000000000000, 0.000000000000000000 ) ) ;
#3505=ORIENTED_EDGE ( 'NONE', *, *, #4960, .F. ) ;
#3510=CARTESIAN_POINT ( 'NONE',  ( 9.877377282685029372E-16, -1.631249998770965659, 2.500000000000000000 ) ) ;
#3518=CARTESIAN_POINT ( 'NONE',  ( 2.256430356250000102, -1.378124999385482941, -2.763330213280484622E-16 ) ) ;
#3528=CARTESIAN_POINT ( 'NONE',  ( -2.499999999999999112, -3.562500000000000444, 1.443375672974065882 ) ) ;
#3529=CARTESIAN_POINT ( 'NONE',  ( 0.6698729810778025762, -3.861153809338631504, 2.500000000000002665 ) ) ;
#3536=CARTESIAN_POINT ( 'NONE',  ( 1.034219503716432668E-14, -4.612500000000000711, -2.500000000000000000 ) ) ;
#3538=ORIENTED_EDGE ( 'NONE', *, *, #3153, .F. ) ;
#3544=VECTOR ( 'NONE', #4149, 1000.000000000000000 ) ;
#3545=FACE_OUTER_BOUND ( 'NONE', #1263, .T. ) ;
#3547=CARTESIAN_POINT ( 'NONE',  ( -2.499999999999999112, -2.212499999999999467, 1.443375672974065882 ) ) ;
#3549=CARTESIAN_POINT ( 'NONE',  ( 5.302876193624534821E-16, -1.687499999999999778, 2.886751345948128655 ) ) ;
#3555=CARTESIAN_POINT ( 'NONE',  ( 2.500000000000000444, -0.6562499987709659033, 1.443375672974063439 ) ) ;
#3558=CARTESIAN_POINT ( 'NONE',  ( 4.996790860652426159E-15, -1.856249998770965748, -2.500000000000000000 ) ) ;
#3561=VERTEX_POINT ( 'NONE', #2181 ) ;
#3563=CARTESIAN_POINT ( 'NONE',  ( -0.6698729810778020211, -4.142403810567665268, -2.500000000000002665 ) ) ;
#3564=CARTESIAN_POINT ( 'NONE',  ( -2.256430356250000102, -0.5906249993854828517, 0.000000000000000000 ) ) ;
#3568=DIRECTION ( 'NONE',  ( 0.000000000000000000, 0.000000000000000000, -1.000000000000000000 ) ) ;
#3570=EDGE_LOOP ( 'NONE', ( #1013, #416 ) ) ;
#3571=EDGE_CURVE ( 'NONE', #9254, #3171, #10280, .T. ) ;
#3574=CARTESIAN_POINT ( 'NONE',  ( 1.128215178124999607, -1.303124999385482985, -1.954126010382871259 ) ) ;
#3575=ORIENTED_EDGE ( 'NONE', *, *, #6979, .F. ) ;
#3581=EDGE_CURVE ( 'NONE', #471, #2983, #610, .T. ) ;
#3584=CYLINDRICAL_SURFACE ( 'NONE', #4979, 2.500000000000000000 ) ;
#3587=CARTESIAN_POINT ( 'NONE',  ( 1.250000000000001110, -2.549999999999999822, 2.165063509461096380 ) ) ;
#3591=DIRECTION ( 'NONE',  ( 0.000000000000000000, -1.000000000000000000, 0.000000000000000000 ) ) ;
#3600=CARTESIAN_POINT ( 'NONE',  ( 3.000000000000000000, -15.00000000000000000, -1.732050807568876749 ) ) ;
#3605=CARTESIAN_POINT ( 'NONE',  ( 1.250000000000001110, -1.199999999999999956, 2.165063509461096380 ) ) ;
#3609=CARTESIAN_POINT ( 'NONE',  ( -1.128215178124998497, -0.6281249993854828295, 1.954126010382872147 ) ) ;
#3616=( NAMED_UNIT ( * ) PLANE_ANGLE_UNIT ( ) SI_UNIT ( $, .RADIAN. ) );
#3621=VERTEX_POINT ( 'NONE', #2236 ) ;
#3622=EDGE_CURVE ( 'NONE', #8050, #1968, #4643, .T. ) ;
#3623=CARTESIAN_POINT ( 'NONE',  ( -1.595409442497313560E-16, -0.2531249993854829405, -2.605501347177161087 ) ) ;
#3630=CARTESIAN_POINT ( 'NONE',  ( 0.000000000000000000, -25.00000000000000000, 0.000000000000000000 ) ) ;
#3632=CARTESIAN_POINT ( 'NONE',  ( 2.256430356250000546, -0.9656249993854827407, 1.302750673588579877 ) ) ;
#3641=CARTESIAN_POINT ( 'NONE',  ( 1.250000000000001110, -0.6937499987709658811, 2.165063509461096380 ) ) ;
#3643=CARTESIAN_POINT ( 'NONE',  ( 0.6698729810778112359, -2.832596189432333933, -2.499999999999996447 ) ) ;
#3651=CARTESIAN_POINT ( 'NONE',  ( -0.6698729810778054627, -0.7513461882033000139, 2.500000000000000000 ) ) ;
#3656=VERTEX_POINT ( 'NONE', #1702 ) ;
#3661=CARTESIAN_POINT ( 'NONE',  ( -1.767625397874844694E-16, -0.5625000000000000000, -2.886751345948128655 ) ) ;
#3664=CARTESIAN_POINT ( 'NONE',  ( -2.256430356250000102, -1.603124999385482807, 0.000000000000000000 ) ) ;
#3671=CYLINDRICAL_SURFACE ( 'NONE', #2891, 2.500000000000000000 ) ;
#3673=CARTESIAN_POINT ( 'NONE',  ( 4.786228327491940187E-16, -1.378124999385482941, 2.605501347177161087 ) ) ;
#3682=CARTESIAN_POINT ( 'NONE',  ( 0.000000000000000000, -15.00000000000000000, -3.464101615137755275 ) ) ;
#3683=CARTESIAN_POINT ( 'NONE',  ( -2.256430356249999214, -2.465624999385482852, 1.302750673588581876 ) ) ;
#3694=FACE_OUTER_BOUND ( 'NONE', #112, .T. ) ;
#3695=CARTESIAN_POINT ( 'NONE',  ( -1.249999999999998224, -2.568749998770965437, 2.165063509461097713 ) ) ;
#3698=DIRECTION ( 'NONE',  ( 0.000000000000000000, 0.000000000000000000, -1.000000000000000000 ) ) ;
#3700=CARTESIAN_POINT ( 'NONE',  ( 2.256430356250000102, -0.8156249993854829405, -2.763330213280484622E-16 ) ) ;
#3710=ORIENTED_EDGE ( 'NONE', *, *, #1823, .F. ) ;
#3711=CARTESIAN_POINT ( 'NONE',  ( -2.499999999999999556, -2.662499999999999645, 1.443375672974065882 ) ) ;
#3713=CARTESIAN_POINT ( 'NONE',  ( 1.249999999999999334, -2.343749998770965792, -2.165063509461096825 ) ) ;
#3715=CARTESIAN_POINT ( 'NONE',  ( -2.256430356250000102, -1.640624999385482896, -1.302750673588580321 ) ) ;
#3716=EDGE_CURVE ( 'NONE', #7134, #3111, #88, .T. ) ;
#3727=CARTESIAN_POINT ( 'NONE',  ( -2.256430356249998770, -1.903124999385482852, 1.302750673588581876 ) ) ;
#3728=CARTESIAN_POINT ( 'NONE',  ( -8.673617379884035472E-16, -15.00000000000000000, 3.464101615137756163 ) ) ;
#3730=PLANE ( 'NONE',  #5585 ) ;
#3739=CARTESIAN_POINT ( 'NONE',  ( -2.256430356250000102, -1.153124999385482852, 0.000000000000000000 ) ) ;
#3744=CARTESIAN_POINT ( 'NONE',  ( 2.256430356250000102, -1.378124999385482941, -2.763330213280484622E-16 ) ) ;
#3748=CARTESIAN_POINT ( 'NONE',  ( 9.877377282685029372E-16, -0.3374999999999999667, 2.500000000000000000 ) ) ;
#3751=CARTESIAN_POINT ( 'NONE',  ( 2.500000000000000000, -4.274999999999999467, -3.061616997868383141E-16 ) ) ;
#3752=CARTESIAN_POINT ( 'NONE',  ( -1.128215178125000273, -0.6656249993854830294, -1.954126010382871259 ) ) ;
#3756=VERTEX_POINT ( 'NONE', #386 ) ;
#3761=VERTEX_POINT ( 'NONE', #8286 ) ;
#3763=DIRECTION ( 'NONE',  ( 0.000000000000000000, -1.000000000000000000, 0.000000000000000000 ) ) ;
#3765=CARTESIAN_POINT ( 'NONE',  ( -1.250000000000000222, -2.774999999999999467, -2.165063509461096825 ) ) ;
#3769=CARTESIAN_POINT ( 'NONE',  ( -2.256430356250000102, -2.990624999385482763, -1.302750673588580321 ) ) ;
#3779=CARTESIAN_POINT ( 'NONE',  ( 2.256430356249999658, -0.3281249993854829516, -1.302750673588581432 ) ) ;
#3782=DIRECTION ( 'NONE',  ( 1.000000000000000000, 0.000000000000000000, -0.000000000000000000 ) ) ;
#3791=( BOUNDED_CURVE ( )  B_SPLINE_CURVE ( 1, ( #3037, #8685 ),
 .UNSPECIFIED., .F., .F. ) 
 B_SPLINE_CURVE_WITH_KNOTS ( ( 2, 2 ),
 ( 0.000000000000000000, 1.000000000000000000 ),
 .UNSPECIFIED. ) 
 CURVE ( )  GEOMETRIC_REPRESENTATION_ITEM ( )  RATIONAL_B_SPLINE_CURVE ( ( 0.9401537613649495473, 0.9401537613649495473 ) ) 
 REPRESENTATION_ITEM ( '' )  );
#3795=CARTESIAN_POINT ( 'NONE',  ( 2.256430356249999658, -4.040624999385483029, -1.302750673588581432 ) ) ;
#3796=EDGE_LOOP ( 'NONE', ( #5326, #1888, #3883, #2068 ) ) ;
#3799=LINE ( 'NONE', #10239, #10070 ) ;
#3802=CARTESIAN_POINT ( 'NONE',  ( -1.595409442497313560E-16, -1.715624999385482852, -2.605501347177161087 ) ) ;
#3805=CARTESIAN_POINT ( 'NONE',  ( 2.500000000000000000, -0.5812499987709658367, -1.443375672974064994 ) ) ;
#3807=CYLINDRICAL_SURFACE ( 'NONE', #3139, 2.500000000000000000 ) ;
#3808=CARTESIAN_POINT ( 'NONE',  ( 1.249999999999999334, -2.849999999999999645, -2.165063509461096825 ) ) ;
#3810=DIRECTION ( 'NONE',  ( 0.000000000000000000, -1.000000000000000000, 0.000000000000000000 ) ) ;
#3811=CARTESIAN_POINT ( 'NONE',  ( 2.256430356250000102, -1.715624999385482852, -2.763330213280484622E-16 ) ) ;
#3812=PRODUCT_DEFINITION_FORMATION_WITH_SPECIFIED_SOURCE ( 'ANY', '', #3022, .NOT_KNOWN. ) ;
#3814=CARTESIAN_POINT ( 'NONE',  ( -2.500000000000000000, -0.8812499987709659921, -1.443375672974064106 ) ) ;
#3817=DIRECTION ( 'NONE',  ( 0.000000000000000000, -1.000000000000000000, 0.000000000000000000 ) ) ;
#3823=CARTESIAN_POINT ( 'NONE',  ( -1.250000000000000222, -4.574999999999999289, -2.165063509461096825 ) ) ;
#3826=CARTESIAN_POINT ( 'NONE',  ( 2.256430356249999658, -3.140624999385482674, -1.302750673588581432 ) ) ;
#3832=EDGE_CURVE ( 'NONE', #10048, #4596, #2640, .T. ) ;
#3833=CYLINDRICAL_SURFACE ( 'NONE', #4638, 2.500000000000000000 ) ;
#3834=CARTESIAN_POINT ( 'NONE',  ( -2.256430356250000102, -1.940624999385482941, 0.000000000000000000 ) ) ;
#3836=CARTESIAN_POINT ( 'NONE',  ( -1.595409442497313560E-16, -2.953124999385482674, -2.605501347177161087 ) ) ;
#3838=VERTEX_POINT ( 'NONE', #8447 ) ;
#3845=ORIENTED_EDGE ( 'NONE', *, *, #8993, .T. ) ;
#3846=CARTESIAN_POINT ( 'NONE',  ( -1.128215178124998497, -4.678124999385482319, 1.954126010382872147 ) ) ;
#3849=CARTESIAN_POINT ( 'NONE',  ( 2.256430356250000102, -0.9281249993854827629, -2.763330213280484622E-16 ) ) ;
#3854=EDGE_CURVE ( 'NONE', #10177, #10048, #9078, .T. ) ;
#3855=CARTESIAN_POINT ( 'NONE',  ( 5.302876193624534821E-16, -1.181249998770965703, 2.886751345948128655 ) ) ;
#3860=CARTESIAN_POINT ( 'NONE',  ( -1.128215178124998497, -0.9656249993854828517, 1.954126010382872147 ) ) ;
#3863=CIRCLE ( 'NONE', #5186, 2.500000000000000000 ) ;
#3864=FACE_OUTER_BOUND ( 'NONE', #1272, .T. ) ;
#3872=DIRECTION ( 'NONE',  ( 0.000000000000000000, -1.000000000000000000, 0.000000000000000000 ) ) ;
#3873=CARTESIAN_POINT ( 'NONE',  ( 2.256430356250000546, -5.015624999385482674, 1.302750673588579877 ) ) ;
#3877=VECTOR ( 'NONE', #3810, 1000.000000000000000 ) ;
#3881=CARTESIAN_POINT ( 'NONE',  ( -2.256430356250000102, -2.428124999385482763, -1.302750673588580321 ) ) ;
#3883=ORIENTED_EDGE ( 'NONE', *, *, #1844, .T. ) ;
#3884=ORIENTED_EDGE ( 'NONE', *, *, #1844, .F. ) ;
#3885=CARTESIAN_POINT ( 'NONE',  ( -1.128215178125000273, -2.015624999385483118, -1.954126010382871259 ) ) ;
#3892=CARTESIAN_POINT ( 'NONE',  ( 3.000000000000000000, -15.00000000000000000, 1.732050807568879192 ) ) ;
#3896=CARTESIAN_POINT ( 'NONE',  ( -1.128215178125000273, -4.828124999385481786, -1.954126010382871259 ) ) ;
#3897=EDGE_LOOP ( 'NONE', ( #7154, #8892, #4802, #4225 ) ) ;
#3901=CARTESIAN_POINT ( 'NONE',  ( -2.256430356249998770, -1.565624999385482941, 1.302750673588581876 ) ) ;
#3907=ORIENTED_EDGE ( 'NONE', *, *, #4748, .F. ) ;
#3908=CARTESIAN_POINT ( 'NONE',  ( -2.499999999999999556, -1.256249998770965659, 1.443375672974065882 ) ) ;
#3914=CARTESIAN_POINT ( 'NONE',  ( -1.128215178124998497, -1.415624999385482807, 1.954126010382872147 ) ) ;
#3920=CARTESIAN_POINT ( 'NONE',  ( -2.500000000000000000, -3.543749998770965526, 0.000000000000000000 ) ) ;
#3924=ORIENTED_EDGE ( 'NONE', *, *, #103, .T. ) ;
#3925=CARTESIAN_POINT ( 'NONE',  ( 1.249999999999999334, -4.649999999999999467, -2.165063509461096825 ) ) ;
#3927=CARTESIAN_POINT ( 'NONE',  ( -1.250000000000000222, -0.4687499987709658478, -2.165063509461096825 ) ) ;
#3928=CARTESIAN_POINT ( 'NONE',  ( -2.256430356250000102, -5.203124999385482674, 0.000000000000000000 ) ) ;
#3937=CARTESIAN_POINT ( 'NONE',  ( -2.256430356249998770, -2.803124999385482763, 1.302750673588581876 ) ) ;
#3940=CARTESIAN_POINT ( 'NONE',  ( 2.256430356250000546, -3.103124999385482585, 1.302750673588579877 ) ) ;
#3942=CARTESIAN_POINT ( 'NONE',  ( 0.000000000000000000, 0.000000000000000000, -2.500000000000000000 ) ) ;
#3945=ORIENTED_EDGE ( 'NONE', *, *, #3581, .F. ) ;
#3949=CARTESIAN_POINT ( 'NONE',  ( 1.128215178125001161, -3.253124999385482496, 1.954126010382870815 ) ) ;
#3951=EDGE_CURVE ( 'NONE', #1383, #4882, #974, .T. ) ;
#3954=CARTESIAN_POINT ( 'NONE',  ( 1.250000000000001110, -4.293749998770965526, 2.165063509461096380 ) ) ;
#3956=CARTESIAN_POINT ( 'NONE',  ( -1.128215178125000273, -3.028124999385482408, -1.954126010382871259 ) ) ;
#3960=CARTESIAN_POINT ( 'NONE',  ( -1.767625397874844694E-16, -3.206249998770965615, -2.886751345948128655 ) ) ;
#3966=CARTESIAN_POINT ( 'NONE',  ( 1.128215178124999607, -3.890624999385482674, -1.954126010382871259 ) ) ;
#3971=ORIENTED_EDGE ( 'NONE', *, *, #8252, .F. ) ;
#3977=CARTESIAN_POINT ( 'NONE',  ( 1.250000000000001110, -3.449999999999999289, 2.165063509461096380 ) ) ;
#3980=CARTESIAN_POINT ( 'NONE',  ( 1.128215178125001161, -4.603124999385482141, 1.954126010382870815 ) ) ;
#3987=EDGE_CURVE ( 'NONE', #9561, #5726, #2024, .T. ) ;
#3990=CARTESIAN_POINT ( 'NONE',  ( -1.128215178125000273, -4.265624999385482674, -1.954126010382871259 ) ) ;
#3993=CARTESIAN_POINT ( 'NONE',  ( -2.256430356249999214, -2.353124999385482585, 1.302750673588581876 ) ) ;
#3996=DIRECTION ( 'NONE',  ( 0.000000000000000000, -1.000000000000000000, 0.000000000000000000 ) ) ;
#4000=ORIENTED_EDGE ( 'NONE', *, *, #2556, .T. ) ;
#4003=CARTESIAN_POINT ( 'NONE',  ( 2.256430356250000102, -4.078124999385482674, -2.763330213280484622E-16 ) ) ;
#4004=ORIENTED_EDGE ( 'NONE', *, *, #8242, .T. ) ;
#4008=CARTESIAN_POINT ( 'NONE',  ( -1.595409442497313560E-16, -4.415624999385482141, -2.605501347177161087 ) ) ;
#4013=CARTESIAN_POINT ( 'NONE',  ( 1.249999999999999334, -3.243749998770965259, -2.165063509461096825 ) ) ;
#4018=CARTESIAN_POINT ( 'NONE',  ( 2.256430356250000546, -4.453124999385482674, 1.302750673588579877 ) ) ;
#4022=CARTESIAN_POINT ( 'NONE',  ( 0.000000000000000000, 0.000000000000000000, -2.500000000000000000 ) ) ;
#4027=VERTEX_POINT ( 'NONE', #6753 ) ;
#4030=CARTESIAN_POINT ( 'NONE',  ( -2.256430356250000102, -3.440624999385482496, -1.302750673588580321 ) ) ;
#4038=CARTESIAN_POINT ( 'NONE',  ( 2.256430356250000102, -4.415624999385482141, -2.763330213280484622E-16 ) ) ;
#4041=CARTESIAN_POINT ( 'NONE',  ( 1.128215178124999607, -1.190624999385482941, -1.954126010382871259 ) ) ;
#4044=DIRECTION ( 'NONE',  ( 0.000000000000000000, 0.000000000000000000, -1.000000000000000000 ) ) ;
#4047=CARTESIAN_POINT ( 'NONE',  ( 0.6698729810778112359, -3.226346188203299992, -2.499999999999996447 ) ) ;
#4049=CARTESIAN_POINT ( 'NONE',  ( 0.000000000000000000, 0.000000000000000000, 0.000000000000000000 ) ) ;
#4052=CARTESIAN_POINT ( 'NONE',  ( 0.6698729810778112359, -5.026346188203299370, -2.499999999999996447 ) ) ;
#4057=CARTESIAN_POINT ( 'NONE',  ( 4.786228327491940187E-16, -2.840624999385482852, 2.605501347177161087 ) ) ;
#4061=VECTOR ( 'NONE', #8403, 1000.000000000000114 ) ;
#4062=CARTESIAN_POINT ( 'NONE',  ( -2.500000000000000000, -2.643749998770965615, 0.000000000000000000 ) ) ;
#4067=CARTESIAN_POINT ( 'NONE',  ( -2.256430356250000102, -3.740624999385482763, 0.000000000000000000 ) ) ;
#4079=CARTESIAN_POINT ( 'NONE',  ( -2.256430356249999658, -5.226765559567681407, -0.8212734853698877568 ) ) ;
#4086=CARTESIAN_POINT ( 'NONE',  ( 2.256430356249999658, -3.928124999385482319, -1.302750673588581432 ) ) ;
#4090=CARTESIAN_POINT ( 'NONE',  ( 1.128215178125001161, -4.940624999385482496, 1.954126010382870815 ) ) ;
#4101=ORIENTED_EDGE ( 'NONE', *, *, #4381, .F. ) ;
#4107=CARTESIAN_POINT ( 'NONE',  ( -1.595409442497313560E-16, -3.065624999385482496, -2.605501347177161087 ) ) ;
#4113=CARTESIAN_POINT ( 'NONE',  ( 1.249999999999999334, -4.593749998770965348, -2.165063509461096825 ) ) ;
#4120=CARTESIAN_POINT ( 'NONE',  ( 2.256430356250000102, -3.065624999385482496, -2.763330213280484622E-16 ) ) ;
#4121=ORIENTED_EDGE ( 'NONE', *, *, #6082, .F. ) ;
#4123=( BOUNDED_CURVE ( )  B_SPLINE_CURVE ( 2, ( #5042, #8018, #2803, #9683, #5988, #5888, #3587, #2523, #1848 ),
 .UNSPECIFIED., .F., .F. ) 
 B_SPLINE_CURVE_WITH_KNOTS ( ( 3, 2, 2, 2, 3 ),
 ( 0.4375000000000000000, 0.4444444444444444198, 0.4583333333333333148, 0.4722222222222222099, 0.4791666666666666852 ),
 .UNSPECIFIED. ) 
 CURVE ( )  GEOMETRIC_REPRESENTATION_ITEM ( )  RATIONAL_B_SPLINE_CURVE ( ( 0.9330127018922194093, 0.9330127018922194093, 1.000000000000000000, 0.8660254037844387076, 1.000000000000000000, 0.8660254037844387076, 1.000000000000000000, 0.9330127018922190762, 0.9330127018922194093 ) ) 
 REPRESENTATION_ITEM ( '' )  );
#4124=CARTESIAN_POINT ( 'NONE',  ( -3.486133158594716510E-16, -2.362499999999999378, -2.500000000000000000 ) ) ;
#4129=CARTESIAN_POINT ( 'NONE',  ( 0.000000000000000000, 0.000000000000000000, 0.000000000000000000 ) ) ;
#4132=DIRECTION ( 'NONE',  ( 0.000000000000000000, -1.000000000000000000, 0.000000000000000000 ) ) ;
#4139=COLOUR_RGB ( '',0.8941176470588234615, 0.8941176470588234615, 0.8941176470588234615 ) ;
#4140=CARTESIAN_POINT ( 'NONE',  ( 1.128215178125001161, -3.590624999385482408, 1.954126010382870815 ) ) ;
#4141=VERTEX_POINT ( 'NONE', #6914 ) ;
#4142=CARTESIAN_POINT ( 'NONE',  ( 1.128215178125001161, -4.040624999385483029, 1.954126010382870815 ) ) ;
#4148=CARTESIAN_POINT ( 'NONE',  ( 2.500000000000000000, -3.337499999999999467, -1.443375672974065438 ) ) ;
#4149=DIRECTION ( 'NONE',  ( 0.000000000000000000, -1.000000000000000000, 0.000000000000000000 ) ) ;
#4154=DIRECTION ( 'NONE',  ( 0.000000000000000000, 0.000000000000000000, 1.000000000000000000 ) ) ;
#4156=CARTESIAN_POINT ( 'NONE',  ( 1.128215178125001161, -4.603124999385482141, 1.954126010382870815 ) ) ;
#4160=CARTESIAN_POINT ( 'NONE',  ( -1.250000000000000222, -4.968749998770965348, -2.165063509461096825 ) ) ;
#4161=ORIENTED_EDGE ( 'NONE', *, *, #9147, .F. ) ;
#4165=CARTESIAN_POINT ( 'NONE',  ( -1.595409442497313560E-16, -3.403124999385483296, -2.605501347177161087 ) ) ;
#4167=ORIENTED_EDGE ( 'NONE', *, *, #3987, .T. ) ;
#4172=DIRECTION ( 'NONE',  ( 0.08715574274765837404, -0.9961946980917455452, 0.000000000000000000 ) ) ;
#4173=DIRECTION ( 'NONE',  ( 0.000000000000000000, 0.000000000000000000, -1.000000000000000000 ) ) ;
#4178=( BOUNDED_CURVE ( )  B_SPLINE_CURVE ( 2, ( #768, #2284, #2968, #4637, #8563, #5484, #5777, #1787, #8872 ),
 .UNSPECIFIED., .F., .F. ) 
 B_SPLINE_CURVE_WITH_KNOTS ( ( 3, 2, 2, 2, 3 ),
 ( 0.3125000000000000000, 0.3194444444444444198, 0.3333333333333333148, 0.3472222222222222099, 0.3541666666666666852 ),
 .UNSPECIFIED. ) 
 CURVE ( )  GEOMETRIC_REPRESENTATION_ITEM ( )  RATIONAL_B_SPLINE_CURVE ( ( 0.9330127018922194093, 0.9330127018922194093, 1.000000000000000000, 0.8660254037844387076, 1.000000000000000000, 0.8660254037844387076, 1.000000000000000000, 0.9330127018922190762, 0.9330127018922194093 ) ) 
 REPRESENTATION_ITEM ( '' )  );
#4180=FACE_OUTER_BOUND ( 'NONE', #9430, .T. ) ;
#4181=CARTESIAN_POINT ( 'NONE',  ( 0.000000000000000000, 0.000000000000000000, -2.500000000000000000 ) ) ;
#4184=ORIENTED_EDGE ( 'NONE', *, *, #3276, .F. ) ;
#4185=CARTESIAN_POINT ( 'NONE',  ( -2.256430356249999214, -3.703124999385482674, 1.302750673588581876 ) ) ;
#4188=CARTESIAN_POINT ( 'NONE',  ( -2.256430356250000102, -0.7406249993854829849, -1.302750673588580321 ) ) ;
#4196=CARTESIAN_POINT ( 'NONE',  ( 1.250000000000001110, -1.593749998770965792, 2.165063509461096380 ) ) ;
#4198=EDGE_CURVE ( 'NONE', #10197, #8050, #9656, .T. ) ;
#4204=CARTESIAN_POINT ( 'NONE',  ( -1.595409442497313560E-16, -0.3656249993854829294, -2.605501347177161087 ) ) ;
#4206=VECTOR ( 'NONE', #1842, 1000.000000000000000 ) ;
#4211=LINE ( 'NONE', #8287, #4206 ) ;
#4214=CARTESIAN_POINT ( 'NONE',  ( 2.500000000000000444, -1.612499999999999822, 1.443375672974063439 ) ) ;
#4218=CARTESIAN_POINT ( 'NONE',  ( -9.703070624755296135E-15, -3.881249998770965881, 2.500000000000000444 ) ) ;
#4219=( GEOMETRIC_REPRESENTATION_CONTEXT ( 3 ) GLOBAL_UNCERTAINTY_ASSIGNED_CONTEXT ( ( #7799 ) ) GLOBAL_UNIT_ASSIGNED_CONTEXT ( ( #6798, #3616, #1099 ) ) REPRESENTATION_CONTEXT ( 'NONE', 'WORKASPACE' ) );
#4224=EDGE_CURVE ( 'NONE', #3171, #957, #11, .T. ) ;
#4225=ORIENTED_EDGE ( 'NONE', *, *, #2364, .T. ) ;
#4228=LINE ( 'NONE', #2708, #8539 ) ;
#4234=ORIENTED_EDGE ( 'NONE', *, *, #9051, .F. ) ;
#4235=CARTESIAN_POINT ( 'NONE',  ( 2.256430356249999658, -3.478124999385482585, -1.302750673588581432 ) ) ;
#4238=CARTESIAN_POINT ( 'NONE',  ( -2.256430356250000102, -0.2531249993854829405, 0.000000000000000000 ) ) ;
#4241=CYLINDRICAL_SURFACE ( 'NONE', #603, 2.500000000000000000 ) ;
#4255=CARTESIAN_POINT ( 'NONE',  ( 1.250000000000001110, -4.743749998770965703, 2.165063509461096380 ) ) ;
#4256=ORIENTED_EDGE ( 'NONE', *, *, #2997, .T. ) ;
#4259=VECTOR ( 'NONE', #8404, 1000.000000000000227 ) ;
#4270=CARTESIAN_POINT ( 'NONE',  ( 9.877377282685029372E-16, -0.7312499987709657479, 2.500000000000000000 ) ) ;
#4284=CARTESIAN_POINT ( 'NONE',  ( 1.128215178125001161, -4.490624999385482319, 1.954126010382870815 ) ) ;
#4304=CARTESIAN_POINT ( 'NONE',  ( 4.786228327491941173E-16, -1.040624999385482585, 2.605501347177161087 ) ) ;
#4310=DIRECTION ( 'NONE',  ( -0.000000000000000000, -1.000000000000000000, -0.000000000000000000 ) ) ;
#4321=ADVANCED_FACE ( 'NONE', ( #949 ), #7127, .T. ) ;
#4332=CARTESIAN_POINT ( 'NONE',  ( -0.6698729810778054627, -4.801346188203300613, 2.500000000000000000 ) ) ;
#4334=CARTESIAN_POINT ( 'NONE',  ( 5.302876193624534821E-16, -2.587499999999999911, 2.886751345948128655 ) ) ;
#4345=CARTESIAN_POINT ( 'NONE',  ( -2.500000000000000000, -4.087500000000000355, -1.443375672974064106 ) ) ;
#4346=ADVANCED_FACE ( 'NONE', ( #7969 ), #8904, .T. ) ;
#4347=CARTESIAN_POINT ( 'NONE',  ( 4.786228327491941173E-16, -0.4781249993854829183, 2.605501347177161087 ) ) ;
#4356=CARTESIAN_POINT ( 'NONE',  ( -2.256430356249999214, -0.6656249993854828073, 1.302750673588581876 ) ) ;
#4362=VECTOR ( 'NONE', #8977, 1000.000000000000114 ) ;
#4366=CARTESIAN_POINT ( 'NONE',  ( 1.249999999999999334, -3.693749998770965437, -2.165063509461096825 ) ) ;
#4368=ORIENTED_EDGE ( 'NONE', *, *, #6527, .T. ) ;
#4371=CARTESIAN_POINT ( 'NONE',  ( -2.500000000000000000, -2.231249998770965970, -1.443375672974064106 ) ) ;
#4372=VECTOR ( 'NONE', #3074, 1000.000000000000000 ) ;
#4375=EDGE_LOOP ( 'NONE', ( #6784, #2279, #9380, #2862 ) ) ;
#4379=FACE_OUTER_BOUND ( 'NONE', #1630, .T. ) ;
#4381=EDGE_CURVE ( 'NONE', #1163, #2926, #2474, .T. ) ;
#4386=CARTESIAN_POINT ( 'NONE',  ( 1.250000000000001110, -1.649999999999999689, 2.165063509461096380 ) ) ;
#4390=CARTESIAN_POINT ( 'NONE',  ( 2.256430356250000546, -0.5156249993854828961, 1.302750673588579877 ) ) ;
#4392=CARTESIAN_POINT ( 'NONE',  ( -1.249999999999998224, -0.8249999999999998446, 2.165063509461097713 ) ) ;
#4402=CARTESIAN_POINT ( 'NONE',  ( -3.486133158594716510E-16, -1.406249998770965570, -2.500000000000000000 ) ) ;
#4409=EDGE_CURVE ( 'NONE', #4798, #9216, #3308, .T. ) ;
#4411=CARTESIAN_POINT ( 'NONE',  ( -1.128215178125000273, -1.678124999385482763, -1.954126010382871259 ) ) ;
#4418=EDGE_LOOP ( 'NONE', ( #3945, #6534, #7835, #2416, #7085, #1246, #10336, #3013 ) ) ;
#4426=CARTESIAN_POINT ( 'NONE',  ( -0.6698729810778043525, -2.286153809338631326, -2.500000000000001332 ) ) ;
#4431=CYLINDRICAL_SURFACE ( 'NONE', #10345, 2.500000000000000000 ) ;
#4432=CARTESIAN_POINT ( 'NONE',  ( 0.000000000000000000, 0.000000000000000000, 0.000000000000000000 ) ) ;
#4433=ORIENTED_EDGE ( 'NONE', *, *, #5829, .T. ) ;
#4436=VERTEX_POINT ( 'NONE', #2420 ) ;
#4437=CARTESIAN_POINT ( 'NONE',  ( 2.500000000000000000, -1.574999999999999734, -3.061616997868383141E-16 ) ) ;
#4440=CARTESIAN_POINT ( 'NONE',  ( 2.256430356250000102, -2.278124999385482852, -2.763330213280484622E-16 ) ) ;
#4449=AXIS2_PLACEMENT_3D ( 'NONE', #7992, #8828, #824 ) ;
#4450=CARTESIAN_POINT ( 'NONE',  ( 1.128215178125001161, -1.790624999385482807, 1.954126010382870815 ) ) ;
#4453=CARTESIAN_POINT ( 'NONE',  ( 1.128215178124999607, -0.7406249993854828739, -1.954126010382871259 ) ) ;
#4456=EDGE_CURVE ( 'NONE', #9475, #4536, #3434, .T. ) ;
#4460=ORIENTED_EDGE ( 'NONE', *, *, #8887, .F. ) ;
#4462=CARTESIAN_POINT ( 'NONE',  ( 1.128215178124999607, -1.753124999385482718, -1.954126010382871259 ) ) ;
#4465=DIRECTION ( 'NONE',  ( -0.08704561088320925122, 0.9949358851208914833, -0.05025580687519627665 ) ) ;
#4466=CARTESIAN_POINT ( 'NONE',  ( 0.6698729810778063509, -4.126346188203299903, -2.500000000000000000 ) ) ;
#4468=CARTESIAN_POINT ( 'NONE',  ( 9.877377282685029372E-16, -3.037499999999999201, 2.500000000000000000 ) ) ;
#4473=ORIENTED_EDGE ( 'NONE', *, *, #6289, .T. ) ;
#4474=EDGE_CURVE ( 'NONE', #8554, #6136, #9945, .T. ) ;
#4477=CARTESIAN_POINT ( 'NONE',  ( 2.256430356249999658, -2.578124999385483118, -1.302750673588581432 ) ) ;
#4484=CARTESIAN_POINT ( 'NONE',  ( -0.6698729810778105698, -3.901346188203299814, 2.499999999999997780 ) ) ;
#4490=CARTESIAN_POINT ( 'NONE',  ( 2.500000000000000444, -2.512500000000000178, 1.443375672974063439 ) ) ;
#4494=CARTESIAN_POINT ( 'NONE',  ( -2.256430356250000102, -1.190624999385482941, -1.302750673588580321 ) ) ;
#4498=CARTESIAN_POINT ( 'NONE',  ( 0.6698729810778087934, -1.932596189432334466, -2.499999999999999112 ) ) ;
#4503=EDGE_LOOP ( 'NONE', ( #2936, #98 ) ) ;
#4504=CARTESIAN_POINT ( 'NONE',  ( -2.256430356249998770, -2.353124999385482585, 1.302750673588581876 ) ) ;
#4507=CARTESIAN_POINT ( 'NONE',  ( -2.256430356250000102, -0.1781249993854829572, -1.302750673588580321 ) ) ;
#4512=ORIENTED_EDGE ( 'NONE', *, *, #5762, .T. ) ;
#4513=( BOUNDED_CURVE ( )  B_SPLINE_CURVE ( 2, ( #8791, #7164, #3927, #6282, #2457 ),
 .UNSPECIFIED., .F., .F. ) 
 B_SPLINE_CURVE_WITH_KNOTS ( ( 3, 2, 3 ),
 ( 0.000000000000000000, 0.01388888888888888812, 0.02083333333333333218 ),
 .UNSPECIFIED. ) 
 CURVE ( )  GEOMETRIC_REPRESENTATION_ITEM ( )  RATIONAL_B_SPLINE_CURVE ( ( 1.000000000000000000, 0.8660254037844387076, 1.000000000000000000, 0.9330127018922194093, 0.9330127018922194093 ) ) 
 REPRESENTATION_ITEM ( '' )  );
#4515=CARTESIAN_POINT ( 'NONE',  ( 4.786228327491941173E-16, -2.390624999385482674, 2.605501347177161087 ) ) ;
#4520=VECTOR ( 'NONE', #5594, 1000.000000000000114 ) ;
#4521=CARTESIAN_POINT ( 'NONE',  ( -1.128215178124998497, -0.6281249993854828295, 1.954126010382872147 ) ) ;
#4525=CARTESIAN_POINT ( 'NONE',  ( 2.500000000000000444, -2.962499999999999911, 1.443375672974063439 ) ) ;
#4527=DIRECTION ( 'NONE',  ( 0.000000000000000000, -1.000000000000000000, 0.000000000000000000 ) ) ;
#4528=CARTESIAN_POINT ( 'NONE',  ( -0.6698729810778020211, -4.536153809338631326, -2.500000000000002665 ) ) ;
#4529=CARTESIAN_POINT ( 'NONE',  ( 1.128215178124999607, -2.090624999385482852, -1.954126010382871259 ) ) ;
#4533=DIRECTION ( 'NONE',  ( 0.000000000000000000, -0.000000000000000000, -1.000000000000000000 ) ) ;
#4536=VERTEX_POINT ( 'NONE', #993 ) ;
#4540=FACE_OUTER_BOUND ( 'NONE', #10031, .T. ) ;
#4543=CARTESIAN_POINT ( 'NONE',  ( 2.500000000000000000, -2.437500000000000000, -1.443375672974064994 ) ) ;
#4547=CARTESIAN_POINT ( 'NONE',  ( 0.6698729810778063509, -3.732596189432333844, -2.500000000000000000 ) ) ;
#4548=CARTESIAN_POINT ( 'NONE',  ( 4.786228327491941173E-16, -2.390624999385482674, 2.605501347177161087 ) ) ;
#4552=AXIS2_PLACEMENT_3D ( 'NONE', #6619, #3591, #344 ) ;
#4555=CARTESIAN_POINT ( 'NONE',  ( -3.000000000000000888, -15.00000000000000000, -1.732050807568877415 ) ) ;
#4556=EDGE_CURVE ( 'NONE', #1808, #2926, #2837, .T. ) ;
#4557=CYLINDRICAL_SURFACE ( 'NONE', #6618, 2.500000000000000000 ) ;
#4558=CARTESIAN_POINT ( 'NONE',  ( -2.256430356250000102, -1.040624999385483029, 0.000000000000000000 ) ) ;
#4561=DIRECTION ( 'NONE',  ( 0.000000000000000000, -0.000000000000000000, 1.000000000000000000 ) ) ;
#4573=CARTESIAN_POINT ( 'NONE',  ( 2.256430356249999658, -3.590624999385481964, -1.302750673588581432 ) ) ;
#4578=CARTESIAN_POINT ( 'NONE',  ( 1.128215178124999607, -0.4031249993854829627, -1.954126010382871259 ) ) ;
#4587=CARTESIAN_POINT ( 'NONE',  ( 2.256430356249999658, -2.128124999385482941, -1.302750673588581432 ) ) ;
#4588=AXIS2_PLACEMENT_3D ( 'NONE', #10332, #4878, #4044 ) ;
#4589=EDGE_CURVE ( 'NONE', #9350, #4614, #8783, .T. ) ;
#4596=VERTEX_POINT ( 'NONE', #5451 ) ;
#4601=CARTESIAN_POINT ( 'NONE',  ( -1.250000000000000222, -4.124999999999999112, -2.165063509461096825 ) ) ;
#4604=CARTESIAN_POINT ( 'NONE',  ( -1.595409442497313560E-16, -3.065624999385482496, -2.605501347177161087 ) ) ;
#4612=CARTESIAN_POINT ( 'NONE',  ( -2.256430356250000102, -1.490624999385482763, 0.000000000000000000 ) ) ;
#4614=VERTEX_POINT ( 'NONE', #6843 ) ;
#4616=CARTESIAN_POINT ( 'NONE',  ( -2.256430356250000102, -2.878124999385482941, -1.302750673588580321 ) ) ;
#4619=ADVANCED_FACE ( 'NONE', ( #8418 ), #2082, .T. ) ;
#4621=ORIENTED_EDGE ( 'NONE', *, *, #2294, .F. ) ;
#4623=EDGE_CURVE ( 'NONE', #1444, #3142, #2023, .T. ) ;
#4628=DIRECTION ( 'NONE',  ( 0.000000000000000000, -1.000000000000000000, 0.000000000000000000 ) ) ;
#4630=CARTESIAN_POINT ( 'NONE',  ( -1.595409442497313560E-16, -4.415624999385482141, -2.605501347177161087 ) ) ;
#4631=VERTEX_POINT ( 'NONE', #1410 ) ;
#4632=DIRECTION ( 'NONE',  ( 0.000000000000000000, -1.000000000000000000, 0.000000000000000000 ) ) ;
#4633=CARTESIAN_POINT ( 'NONE',  ( 0.6698729810778065730, -0.1325961894323341994, -2.499999999999999556 ) ) ;
#4634=AXIS2_PLACEMENT_3D ( 'NONE', #5085, #8976, #4989 ) ;
#4635=CARTESIAN_POINT ( 'NONE',  ( -2.256430356250000102, -1.190624999385482941, -1.302750673588580321 ) ) ;
#4637=CARTESIAN_POINT ( 'NONE',  ( -2.499999999999999112, -1.762499999999999734, 1.443375672974065882 ) ) ;
#4638=AXIS2_PLACEMENT_3D ( 'NONE', #6907, #3051, #10105 ) ;
#4639=CARTESIAN_POINT ( 'NONE',  ( -2.500000000000000000, -1.781249998770965570, -1.443375672974064106 ) ) ;
#4642=ORIENTED_EDGE ( 'NONE', *, *, #5762, .F. ) ;
#4643=LINE ( 'NONE', #7836, #7534 ) ;
#4644=( BOUNDED_CURVE ( )  B_SPLINE_CURVE ( 2, ( #7384, #1785, #3713, #6896, #7338, #222, #1882, #5027, #9065 ),
 .UNSPECIFIED., .F., .T. ) 
 B_SPLINE_CURVE_WITH_KNOTS ( ( 3, 2, 2, 2, 3 ),
 ( 0.3541666666666666852, 0.3611111111111111049, 0.3750000000000000000, 0.3888888888888888951, 0.3958333333333333703 ),
 .UNSPECIFIED. ) 
 CURVE ( )  GEOMETRIC_REPRESENTATION_ITEM ( )  RATIONAL_B_SPLINE_CURVE ( ( 0.9330127018922194093, 0.9330127018922196314, 1.000000000000000000, 0.8660254037844387076, 1.000000000000000000, 0.8660254037844387076, 1.000000000000000000, 0.9330127018922190762, 0.9330127018922194093 ) ) 
 REPRESENTATION_ITEM ( '' )  );
#4645=CARTESIAN_POINT ( 'NONE',  ( -2.256430356250000102, -1.528124999385482630, -1.302750673588580321 ) ) ;
#4648=FACE_OUTER_BOUND ( 'NONE', #3796, .T. ) ;
#4656=ORIENTED_EDGE ( 'NONE', *, *, #3264, .F. ) ;
#4659=CARTESIAN_POINT ( 'NONE',  ( 0.6698729810778025762, -3.917403810567665623, 2.500000000000002665 ) ) ;
#4660=CARTESIAN_POINT ( 'NONE',  ( 2.256430356250000102, -1.828124999385482674, -2.763330213280484622E-16 ) ) ;
#4667=DIRECTION ( 'NONE',  ( 0.8660254037844385966, 0.000000000000000000, -0.5000000000000000000 ) ) ;
#4668=DIRECTION ( 'NONE',  ( 0.000000000000000000, 0.000000000000000000, -1.000000000000000000 ) ) ;
#4669=CARTESIAN_POINT ( 'NONE',  ( 1.128215178124999607, -2.090624999385482852, -1.954126010382871259 ) ) ;
#4673=CARTESIAN_POINT ( 'NONE',  ( -1.128215178125000273, -1.565624999385482941, -1.954126010382871259 ) ) ;
#4684=CARTESIAN_POINT ( 'NONE',  ( 4.786228327491941173E-16, -4.190624999385482496, 2.605501347177161087 ) ) ;
#4686=EDGE_CURVE ( 'NONE', #1838, #7872, #4513, .T. ) ;
#4690=CARTESIAN_POINT ( 'NONE',  ( -1.128215178124998497, -2.428124999385482763, 1.954126010382872147 ) ) ;
#4693=CARTESIAN_POINT ( 'NONE',  ( 1.250000000000001110, -2.493749998770965703, 2.165063509461096380 ) ) ;
#4699=CARTESIAN_POINT ( 'NONE',  ( 2.256430356250000102, -2.165624999385483029, -2.763330213280484622E-16 ) ) ;
#4703=VERTEX_POINT ( 'NONE', #9976 ) ;
#4707=CARTESIAN_POINT ( 'NONE',  ( 2.500000000000000444, -3.862499999999999822, 1.443375672974063439 ) ) ;
#4709=CARTESIAN_POINT ( 'NONE',  ( -1.128215178125000273, -4.828124999385481786, -1.954126010382871259 ) ) ;
#4717=CARTESIAN_POINT ( 'NONE',  ( -2.256430356250000102, -3.740624999385482763, 0.000000000000000000 ) ) ;
#4721=CARTESIAN_POINT ( 'NONE',  ( 2.256430356250000102, -3.065624999385482496, -2.763330213280484622E-16 ) ) ;
#4726=EDGE_CURVE ( 'NONE', #2231, #957, #350, .T. ) ;
#4728=CARTESIAN_POINT ( 'NONE',  ( 1.249999999999999334, -3.299999999999999378, -2.165063509461096825 ) ) ;
#4731=CARTESIAN_POINT ( 'NONE',  ( 1.128215178125001161, -3.703124999385482230, 1.954126010382870815 ) ) ;
#4736=CARTESIAN_POINT ( 'NONE',  ( -1.128215178125000273, -1.678124999385482763, -1.954126010382871259 ) ) ;
#4741=CARTESIAN_POINT ( 'NONE',  ( -1.249999999999998224, -2.118749998770965703, 2.165063509461097713 ) ) ;
#4742=ORIENTED_EDGE ( 'NONE', *, *, #3277, .T. ) ;
#4744=CARTESIAN_POINT ( 'NONE',  ( -9.703070624755296135E-15, -4.331249998770966059, 2.500000000000000444 ) ) ;
#4745=CARTESIAN_POINT ( 'NONE',  ( 2.256430356249999658, -3.478124999385482585, -1.302750673588581432 ) ) ;
#4747=ORIENTED_EDGE ( 'NONE', *, *, #2997, .F. ) ;
#4748=EDGE_CURVE ( 'NONE', #4798, #3656, #7776, .T. ) ;
#4755=CARTESIAN_POINT ( 'NONE',  ( 2.500000000000000000, -3.337499999999999467, -1.443375672974064994 ) ) ;
#4757=CARTESIAN_POINT ( 'NONE',  ( 2.256430356249999658, -4.040624999385483029, -1.302750673588581432 ) ) ;
#4766=CARTESIAN_POINT ( 'NONE',  ( 2.256430356249999658, -3.478124999385482585, -1.302750673588581432 ) ) ;
#4771=CARTESIAN_POINT ( 'NONE',  ( 2.256430356249999658, -1.678124999385482541, -1.302750673588581432 ) ) ;
#4780=CARTESIAN_POINT ( 'NONE',  ( 4.786228327491941173E-16, -3.740624999385482319, 2.605501347177161087 ) ) ;
#4786=CARTESIAN_POINT ( 'NONE',  ( -2.256430356250000102, -2.953124999385482674, 0.000000000000000000 ) ) ;
#4790=CARTESIAN_POINT ( 'NONE',  ( -2.499999999999999556, -2.606249998770965526, 1.443375672974065882 ) ) ;
#4791=VECTOR ( 'NONE', #1602, 1000.000000000000114 ) ;
#4792=CARTESIAN_POINT ( 'NONE',  ( 0.6698729810778075722, -1.161153809338631770, 2.499999999999999556 ) ) ;
#4795=CARTESIAN_POINT ( 'NONE',  ( 1.128215178124999607, -4.340624999385482852, -1.954126010382871259 ) ) ;
#4798=VERTEX_POINT ( 'NONE', #6939 ) ;
#4799=LINE ( 'NONE', #7996, #254 ) ;
#4802=ORIENTED_EDGE ( 'NONE', *, *, #8074, .T. ) ;
#4804=CARTESIAN_POINT ( 'NONE',  ( 1.250000000000001110, -2.043749998770965970, 2.165063509461096380 ) ) ;
#4805=EDGE_CURVE ( 'NONE', #2167, #5722, #10081, .T. ) ;
#4809=CARTESIAN_POINT ( 'NONE',  ( 2.500000000000000000, -4.724999999999998757, -3.061616997868383141E-16 ) ) ;
#4810=CARTESIAN_POINT ( 'NONE',  ( 2.256430356250000102, -3.178124999385482319, -2.763330213280484622E-16 ) ) ;
#4812=CARTESIAN_POINT ( 'NONE',  ( -2.256430356249999214, -3.815624999385482941, 1.302750673588581876 ) ) ;
#4821=CARTESIAN_POINT ( 'NONE',  ( 2.256430356250000102, -2.615624999385482763, -2.763330213280484622E-16 ) ) ;
#4824=CARTESIAN_POINT ( 'NONE',  ( 1.128215178125001161, -1.790624999385482807, 1.954126010382870815 ) ) ;
#4833=ORIENTED_EDGE ( 'NONE', *, *, #5449, .T. ) ;
#4837=CARTESIAN_POINT ( 'NONE',  ( 1.249999999999999334, -4.143749998770966059, -2.165063509461096825 ) ) ;
#4839=CARTESIAN_POINT ( 'NONE',  ( -2.256430356250000102, -4.340624999385482852, -1.302750673588580321 ) ) ;
#4845=CARTESIAN_POINT ( 'NONE',  ( 2.500000000000000000, -1.931249998770965481, -1.443375672974064994 ) ) ;
#4850=CARTESIAN_POINT ( 'NONE',  ( 2.256430356250000546, -3.553124999385482763, 1.302750673588579877 ) ) ;
#4852=ORIENTED_EDGE ( 'NONE', *, *, #4686, .F. ) ;
#4856=( BOUNDED_CURVE ( )  B_SPLINE_CURVE ( 2, ( #7443, #6570, #5784, #8193, #5090, #4214, #5743, #3287, #5039 ),
 .UNSPECIFIED., .F., .T. ) 
 B_SPLINE_CURVE_WITH_KNOTS ( ( 3, 2, 2, 2, 3 ),
 ( 0.2708333333333333703, 0.2777777777777777901, 0.2916666666666666852, 0.3055555555555555802, 0.3125000000000000000 ),
 .UNSPECIFIED. ) 
 CURVE ( )  GEOMETRIC_REPRESENTATION_ITEM ( )  RATIONAL_B_SPLINE_CURVE ( ( 0.9330127018922194093, 0.9330127018922196314, 1.000000000000000000, 0.8660254037844387076, 1.000000000000000000, 0.8660254037844387076, 1.000000000000000000, 0.9330127018922194093, 0.9330127018922194093 ) ) 
 REPRESENTATION_ITEM ( '' )  );
#4857=CARTESIAN_POINT ( 'NONE',  ( -0.6698729810778105698, -3.507596189432333311, 2.499999999999997780 ) ) ;
#4864=CARTESIAN_POINT ( 'NONE',  ( 1.128215178125001161, -5.053124999385482319, 1.954126010382870815 ) ) ;
#4868=CARTESIAN_POINT ( 'NONE',  ( 0.6698729810778050187, -2.117403810567665801, 2.500000000000000444 ) ) ;
#4871=FACE_OUTER_BOUND ( 'NONE', #409, .T. ) ;
#4872=DIRECTION ( 'NONE',  ( 0.9961946980917455452, -0.08715574274765837404, 0.000000000000000000 ) ) ;
#4873=CARTESIAN_POINT ( 'NONE',  ( -2.256430356250000102, -3.290624999385482585, 0.000000000000000000 ) ) ;
#4876=CARTESIAN_POINT ( 'NONE',  ( -2.256430356250000102, -4.678124999385483207, -1.302750673588580321 ) ) ;
#4878=DIRECTION ( 'NONE',  ( 0.000000000000000000, -1.000000000000000000, 0.000000000000000000 ) ) ;
#4882=VERTEX_POINT ( 'NONE', #6604 ) ;
#4891=CARTESIAN_POINT ( 'NONE',  ( -1.128215178124998497, -4.678124999385482319, 1.954126010382872147 ) ) ;
#4896=CARTESIAN_POINT ( 'NONE',  ( -2.499999999999999556, -4.406249998770965348, 1.443375672974065882 ) ) ;
#4899=CARTESIAN_POINT ( 'NONE',  ( 1.034219503716432668E-14, -3.262500000000000178, -2.500000000000000000 ) ) ;
#4900=EDGE_CURVE ( 'NONE', #7872, #6035, #8331, .T. ) ;
#4902=CARTESIAN_POINT ( 'NONE',  ( -2.256430356249999214, -3.253124999385482941, 1.302750673588581876 ) ) ;
#4905=CARTESIAN_POINT ( 'NONE',  ( 0.000000000000000000, 0.000000000000000000, -2.500000000000000000 ) ) ;
#4911=CARTESIAN_POINT ( 'NONE',  ( 1.128215178124999607, -0.2906249993854829738, -1.954126010382871259 ) ) ;
#4918=CARTESIAN_POINT ( 'NONE',  ( 2.256430356249999658, -4.378124999385483385, -1.302750673588581432 ) ) ;
#4921=CARTESIAN_POINT ( 'NONE',  ( -2.256430356250000102, -5.090624999385482852, 0.000000000000000000 ) ) ;
#4925=VECTOR ( 'NONE', #6349, 1000.000000000000000 ) ;
#4935=CARTESIAN_POINT ( 'NONE',  ( -1.128215178124998497, -4.228124999385482141, 1.954126010382872147 ) ) ;
#4939=CARTESIAN_POINT ( 'NONE',  ( -1.249999999999998224, -5.268749998770966059, 2.165063509461097713 ) ) ;
#4941=DIRECTION ( 'NONE',  ( -0.000000000000000000, -1.000000000000000000, -0.000000000000000000 ) ) ;
#4944=CARTESIAN_POINT ( 'NONE',  ( -1.128215178125000273, -2.915624999385482585, -1.954126010382871259 ) ) ;
#4945=ORIENTED_EDGE ( 'NONE', *, *, #2183, .T. ) ;
#4947=VECTOR ( 'NONE', #10168, 1000.000000000000000 ) ;
#4948=DIRECTION ( 'NONE',  ( 0.000000000000000000, 0.000000000000000000, -1.000000000000000000 ) ) ;
#4955=FACE_OUTER_BOUND ( 'NONE', #2093, .T. ) ;
#4957=CARTESIAN_POINT ( 'NONE',  ( 0.000000000000000000, 0.000000000000000000, 0.000000000000000000 ) ) ;
#4958=CARTESIAN_POINT ( 'NONE',  ( 2.500000000000000444, -4.706249998770965171, 1.443375672974063439 ) ) ;
#4959=LINE ( 'NONE', #4181, #6239 ) ;
#4960=EDGE_CURVE ( 'NONE', #6136, #8554, #5776, .T. ) ;
#4962=CARTESIAN_POINT ( 'NONE',  ( 1.034219503716432668E-14, -5.006249998770964993, -2.500000000000000000 ) ) ;
#4963=CARTESIAN_POINT ( 'NONE',  ( -1.728534191064767578, -5.141148192311419507, -1.450395636689028711 ) ) ;
#4964=SURFACE_STYLE_FILL_AREA ( #3350 ) ;
#4966=( BOUNDED_CURVE ( )  B_SPLINE_CURVE ( 2, ( #7516, #206, #9933, #3547, #8207, #6735, #253, #5163, #8996 ),
 .UNSPECIFIED., .F., .F. ) 
 B_SPLINE_CURVE_WITH_KNOTS ( ( 3, 2, 2, 2, 3 ),
 ( 0.3958333333333333703, 0.4027777777777777901, 0.4166666666666666852, 0.4305555555555555802, 0.4375000000000000000 ),
 .UNSPECIFIED. ) 
 CURVE ( )  GEOMETRIC_REPRESENTATION_ITEM ( )  RATIONAL_B_SPLINE_CURVE ( ( 0.9330127018922194093, 0.9330127018922196314, 1.000000000000000000, 0.8660254037844387076, 1.000000000000000000, 0.8660254037844387076, 1.000000000000000000, 0.9330127018922194093, 0.9330127018922194093 ) ) 
 REPRESENTATION_ITEM ( '' )  );
#4970=CARTESIAN_POINT ( 'NONE',  ( -2.500000000000000000, -1.349999999999999867, 0.000000000000000000 ) ) ;
#4976=CARTESIAN_POINT ( 'NONE',  ( 2.500000000000000444, -1.556249998770966148, 1.443375672974063439 ) ) ;
#4979=AXIS2_PLACEMENT_3D ( 'NONE', #10072, #9347, #8395 ) ;
#4980=CARTESIAN_POINT ( 'NONE',  ( 2.256430356250000102, -3.628124999385482496, -2.763330213280484622E-16 ) ) ;
#4985=CARTESIAN_POINT ( 'NONE',  ( -1.249999999999998224, -3.918749998770965082, 2.165063509461097713 ) ) ;
#4988=DIRECTION ( 'NONE',  ( 0.000000000000000000, -1.000000000000000000, 0.000000000000000000 ) ) ;
#4989=DIRECTION ( 'NONE',  ( 0.000000000000000000, -0.000000000000000000, -1.000000000000000000 ) ) ;
#4994=CARTESIAN_POINT ( 'NONE',  ( -3.486133158594716510E-16, -3.712499999999999467, -2.500000000000000000 ) ) ;
#4995=LINE ( 'NONE', #287, #1115 ) ;
#4997=CYLINDRICAL_SURFACE ( 'NONE', #5416, 2.500000000000000000 ) ;
#5007=DIRECTION ( 'NONE',  ( 0.000000000000000000, 0.000000000000000000, -1.000000000000000000 ) ) ;
#5008=CARTESIAN_POINT ( 'NONE',  ( 1.128215178125001161, -4.940624999385482496, 1.954126010382870815 ) ) ;
#5012=CARTESIAN_POINT ( 'NONE',  ( 1.128215178124999607, -3.890624999385482674, -1.954126010382871259 ) ) ;
#5019=CARTESIAN_POINT ( 'NONE',  ( -0.6698729810778043525, -1.442403810567665756, -2.500000000000001332 ) ) ;
#5027=CARTESIAN_POINT ( 'NONE',  ( 0.6698729810778050187, -2.511153809338630971, 2.500000000000000444 ) ) ;
#5032=CARTESIAN_POINT ( 'NONE',  ( 2.256430356250000102, -0.4781249993854829183, -2.763330213280484622E-16 ) ) ;
#5039=CARTESIAN_POINT ( 'NONE',  ( 9.877377282685029372E-16, -1.687499999999999778, 2.500000000000000000 ) ) ;
#5040=DIRECTION ( 'NONE',  ( 0.000000000000000000, -1.000000000000000000, 0.000000000000000000 ) ) ;
#5042=CARTESIAN_POINT ( 'NONE',  ( -3.486133158594716510E-16, -2.362499999999999378, -2.500000000000000000 ) ) ;
#5043=MECHANICAL_DESIGN_GEOMETRIC_PRESENTATION_REPRESENTATION('',(#9740),#4219);
#5049=DIRECTION ( 'NONE',  ( 0.000000000000000000, -1.000000000000000000, 0.000000000000000000 ) ) ;
#5055=AXIS2_PLACEMENT_3D ( 'NONE', #9842, #4154, #9744 ) ;
#5059=CARTESIAN_POINT ( 'NONE',  ( -0.6698729810778020211, -4.986153809338630616, -2.500000000000002665 ) ) ;
#5061=CARTESIAN_POINT ( 'NONE',  ( -1.128215178125000273, -4.715624999385481964, -1.954126010382871259 ) ) ;
#5062=SHAPE_REPRESENTATION_RELATIONSHIP ( 'NONE' , 'NONE' ,  #9736, #5870 ) ;
#5072=CARTESIAN_POINT ( 'NONE',  ( 2.500000000000000000, -1.481249998770965970, -1.443375672974065438 ) ) ;
#5081=CARTESIAN_POINT ( 'NONE',  ( 1.250000000000001110, -4.293749998770965526, 2.165063509461096380 ) ) ;
#5085=CARTESIAN_POINT ( 'NONE',  ( 0.000000000000000000, 0.000000000000000000, 0.000000000000000000 ) ) ;
#5087=DIRECTION ( 'NONE',  ( -0.8660254037844387076, -0.000000000000000000, 0.4999999999999997780 ) ) ;
#5088=CARTESIAN_POINT ( 'NONE',  ( 0.000000000000000000, -25.00000000000000000, 0.000000000000000000 ) ) ;
#5090=CARTESIAN_POINT ( 'NONE',  ( 2.500000000000000000, -1.574999999999999734, -3.061616997868383141E-16 ) ) ;
#5099=CARTESIAN_POINT ( 'NONE',  ( -1.249999999999998224, -4.424999999999998934, 2.165063509461097713 ) ) ;
#5104=CARTESIAN_POINT ( 'NONE',  ( 3.061616997868383141E-16, -15.00000000000000000, 2.500000000000000000 ) ) ;
#5105=CARTESIAN_POINT ( 'NONE',  ( 1.249999999999999334, -4.593749998770965348, -2.165063509461096825 ) ) ;
#5106=CARTESIAN_POINT ( 'NONE',  ( -1.249999999999998224, -0.3749999999999999445, 2.165063509461097713 ) ) ;
#5109=DIRECTION ( 'NONE',  ( 0.000000000000000000, 0.000000000000000000, -1.000000000000000000 ) ) ;
#5111=AXIS2_PLACEMENT_3D ( 'NONE', #9852, #971, #7346 ) ;
#5112=CIRCLE ( 'NONE', #7005, 2.062556682370379590 ) ;
#5113=CARTESIAN_POINT ( 'NONE',  ( 1.249999999999999334, -0.5999999999999999778, -2.165063509461096825 ) ) ;
#5126=CARTESIAN_POINT ( 'NONE',  ( -9.703070624755296135E-15, -3.937500000000000888, 2.500000000000000444 ) ) ;
#5136=CARTESIAN_POINT ( 'NONE',  ( 2.256430356249999658, -1.340624999385482852, -1.302750673588581432 ) ) ;
#5143=ADVANCED_FACE ( 'NONE', ( #104 ), #8793, .T. ) ;
#5146=CARTESIAN_POINT ( 'NONE',  ( -2.500000000000000000, -0.8437499987709659033, 0.000000000000000000 ) ) ;
#5152=CARTESIAN_POINT ( 'NONE',  ( -2.500000000000000000, -4.949999999999999289, 0.000000000000000000 ) ) ;
#5158=LINE ( 'NONE', #3089, #4520 ) ;
#5163=CARTESIAN_POINT ( 'NONE',  ( -0.6698729810778069060, -2.342403810567665445, -2.500000000000000000 ) ) ;
#5164=ORIENTED_EDGE ( 'NONE', *, *, #9274, .F. ) ;
#5165=CARTESIAN_POINT ( 'NONE',  ( -2.499999999999999556, -1.312500000000000000, 1.443375672974065882 ) ) ;
#5180=FACE_OUTER_BOUND ( 'NONE', #5911, .T. ) ;
#5182=CARTESIAN_POINT ( 'NONE',  ( -0.6698729810778054627, -1.651346188203300036, 2.500000000000000000 ) ) ;
#5186=AXIS2_PLACEMENT_3D ( 'NONE', #830, #1507, #2243 ) ;
#5190=CARTESIAN_POINT ( 'NONE',  ( 2.256430356250000102, -2.728124999385482585, -2.763330213280484622E-16 ) ) ;
#5194=CARTESIAN_POINT ( 'NONE',  ( 2.781278341185189795, -20.00000000000000000, 1.353213781785882031 ) ) ;
#5197=CARTESIAN_POINT ( 'NONE',  ( -1.767625397874844694E-16, -0.5062499987709657701, -2.886751345948128655 ) ) ;
#5202=CARTESIAN_POINT ( 'NONE',  ( -1.915120254295647362, -5.000523192925935945, -1.606958123781256464 ) ) ;
#5208=DIRECTION ( 'NONE',  ( 0.000000000000000000, -1.000000000000000000, 0.000000000000000000 ) ) ;
#5210=CARTESIAN_POINT ( 'NONE',  ( -3.061616997868383634E-16, -20.00000000000000000, 2.500000000000000444 ) ) ;
#5217=CARTESIAN_POINT ( 'NONE',  ( -1.767625397874844694E-16, -2.362499999999999822, -2.886751345948128655 ) ) ;
#5218=CARTESIAN_POINT ( 'NONE',  ( 1.250000000000001110, -3.899999999999999911, 2.165063509461096380 ) ) ;
#5219=CARTESIAN_POINT ( 'NONE',  ( -1.128215178125000273, -2.578124999385482674, -1.954126010382871259 ) ) ;
#5222=CARTESIAN_POINT ( 'NONE',  ( 0.6698729810778075722, -0.7111538093386315929, 2.499999999999999556 ) ) ;
#5225=CARTESIAN_POINT ( 'NONE',  ( 4.996790860652426159E-15, -1.912499999999999867, -2.500000000000000000 ) ) ;
#5229=CARTESIAN_POINT ( 'NONE',  ( -2.256430356249998770, -1.453124999385482896, 1.302750673588581876 ) ) ;
#5230=CARTESIAN_POINT ( 'NONE',  ( -1.915118561403101660, -5.394273269507307234, -1.606960141313192203 ) ) ;
#5232=CARTESIAN_POINT ( 'NONE',  ( 1.128215178125001161, -0.8906249993854827851, 1.954126010382870815 ) ) ;
#5239=( BOUNDED_SURFACE ( )  B_SPLINE_SURFACE ( 1, 2, ( 
 ( #4238, #312, #2717, #9101, #7419, #9155, #8368, #4390, #7575, #413, #3609, #9732, #5764, #4188, #3045, #9250, #525, #10039, #2198, #8476, #9426, #5452, #7850, #6225, #6955, #4494, #2253, #6844, #10158, #8643, #8531, #7007, #1467, #10211, #1250, #7686, #3664, #3715, #8590, #5341, #680, #2083, #4660, #5398, #6792, #9991, #10094, #468, #5277, #1356, #7796, #2875, #6059, #9369, #4440, #2025, #2827, #4548, #6007, #7742, #1304, #9200, #5219, #576, #6898, #2991, #8419, #2140, #7628, #2933, #6115, #1411, #9308, #3769, #6171, #4604, #627, #3826, #4810, #8054, #5703, #8743, #1567, #46, #6336, #4030, #2354, #6484, #7115, #3199, #3293, #8007, #9479, #6433, #6381, #4812, #9674, #10315, #838, #7059, #2458, #4757, #3152, #1618, #7212, #5506, #2512, #9530, #7955, #5551, #3246, #788, #2306, #8695, #9626, #2406, #3980, #5654, #1516, #9574, #8844, #3099, #4709, #7902, #735, #1670, #7165, #3873, #4864, #5602, #889, #8792, #3928, #4079, #7261 ),
 ( #6283, #102, #8890, #1715, #4911, #8108, #10267, #8572, #719, #8680, #9353, #8629, #7669, #5381, #3752, #2124, #6268, #6882, #3700, #9465, #666, #10079, #3860, #10253, #611, #7046, #5323, #10199, #2976, #506, #7837, #2341, #6323, #1452, #3914, #2915, #6098, #4645, #7780, #7099, #1342, #1398, #3811, #6995, #9516, #3084, #2293, #9291, #3034, #5490, #8513, #1503, #4529, #4587, #4699, #1287, #7887, #10304, #6210, #7725, #560, #6938, #10139, #3136, #9408, #4477, #8458, #6156, #2182, #2237, #5439, #975, #3284, #3186, #4944, #7994, #7304, #8043, #4120, #9565, #7251, #30, #7942, #4902, #9756, #3371, #5692, #4165, #775, #4745, #1703, #4850, #7349, #8778, #5640, #876, #4067, #6565, #141, #3331, #3966, #89, #8097, #2396, #926, #5592, #8831, #5739, #8732, #8881, #9709, #1659, #4795, #1605, #826, #4018, #186, #6473, #1555, #2547, #6519, #8928, #5541, #9663, #7152, #2498, #6371, #8146, #7202, #3234, #1748, #10355, #6422, #9612, #2445 ) ),
 .UNSPECIFIED., .F., .F., .F. ) 
 B_SPLINE_SURFACE_WITH_KNOTS ( ( 2, 2 ),
 ( 3, 2, 2, 2, 2, 2, 2, 2, 2, 2, 2, 2, 2, 2, 2, 2, 2, 2, 2, 2, 2, 2, 2, 2, 2, 2, 2, 2, 2, 2, 2, 2, 2, 2, 2, 2, 2, 2, 2, 2, 2, 2, 2, 2, 2, 2, 2, 2, 2, 2, 2, 2, 2, 2, 2, 2, 2, 2, 2, 2, 2, 2, 2, 2, 2, 2, 2, 3 ),
 ( 0.000000000000000000, 1.000000000000000000 ),
 ( 0.000000000000000000, 0.01388888888888888812, 0.02777777777777777624, 0.04166666666666666435, 0.05555555555555555247, 0.06944444444444444753, 0.08333333333333332871, 0.09722222222222222376, 0.1111111111111111049, 0.1250000000000000000, 0.1388888888888888951, 0.1527777777777777901, 0.1666666666666666574, 0.1805555555555555525, 0.1944444444444444475, 0.2083333333333333426, 0.2222222222222222099, 0.2361111111111111049, 0.2500000000000000000, 0.2638888888888888951, 0.2777777777777777901, 0.2916666666666666852, 0.3055555555555555802, 0.3194444444444444198, 0.3333333333333333148, 0.3472222222222222099, 0.3611111111111111049, 0.3750000000000000000, 0.3888888888888888951, 0.4027777777777777901, 0.4166666666666666852, 0.4305555555555555802, 0.4444444444444444198, 0.4583333333333333148, 0.4722222222222222099, 0.4861111111111111049, 0.5000000000000000000, 0.5138888888888888395, 0.5277777777777777901, 0.5416666666666666297, 0.5555555555555555802, 0.5694444444444444198, 0.5833333333333333703, 0.5972222222222222099, 0.6111111111111111605, 0.6250000000000000000, 0.6388888888888888395, 0.6527777777777777901, 0.6666666666666666297, 0.6805555555555555802, 0.6944444444444444198, 0.7083333333333333703, 0.7222222222222222099, 0.7361111111111111605, 0.7500000000000000000, 0.7638888888888888395, 0.7777777777777777901, 0.7916666666666666297, 0.8055555555555555802, 0.8194444444444444198, 0.8333333333333333703, 0.8472222222222222099, 0.8611111111111111605, 0.8750000000000000000, 0.8888888888888888395, 0.9027777777777777901, 0.9166666666666666297, 0.9258785565094815873 ),
 .UNSPECIFIED. ) 
 GEOMETRIC_REPRESENTATION_ITEM ( )  RATIONAL_B_SPLINE_SURFACE ( (
 ( 1.000000000000000000, 0.8660254037844387076, 1.000000000000000000, 0.8660254037844387076, 1.000000000000000000, 0.8660254037844387076, 1.000000000000000000, 0.8660254037844387076, 1.000000000000000000, 0.8660254037844387076, 1.000000000000000000, 0.8660254037844387076, 1.000000000000000000, 0.8660254037844387076, 1.000000000000000000, 0.8660254037844387076, 1.000000000000000000, 0.8660254037844387076, 1.000000000000000000, 0.8660254037844387076, 1.000000000000000000, 0.8660254037844387076, 1.000000000000000000, 0.8660254037844387076, 1.000000000000000000, 0.8660254037844387076, 1.000000000000000000, 0.8660254037844387076, 1.000000000000000000, 0.8660254037844387076, 1.000000000000000000, 0.8660254037844387076, 1.000000000000000000, 0.8660254037844387076, 1.000000000000000000, 0.8660254037844387076, 1.000000000000000000, 0.8660254037844387076, 1.000000000000000000, 0.8660254037844387076, 1.000000000000000000, 0.8660254037844387076, 1.000000000000000000, 0.8660254037844387076, 1.000000000000000000, 0.8660254037844387076, 1.000000000000000000, 0.8660254037844387076, 1.000000000000000000, 0.8660254037844387076, 1.000000000000000000, 0.8660254037844387076, 1.000000000000000000, 0.8660254037844387076, 1.000000000000000000, 0.8660254037844387076, 1.000000000000000000, 0.8660254037844387076, 1.000000000000000000, 0.8660254037844387076, 1.000000000000000000, 0.8660254037844387076, 1.000000000000000000, 0.8660254037844387076, 1.000000000000000000, 0.8660254037844387076, 1.000000000000000000, 0.8660254037844387076, 1.000000000000000000, 0.8660254037844387076, 1.000000000000000000, 0.8660254037844387076, 1.000000000000000000, 0.8660254037844387076, 1.000000000000000000, 0.8660254037844387076, 1.000000000000000000, 0.8660254037844387076, 1.000000000000000000, 0.8660254037844387076, 1.000000000000000000, 0.8660254037844387076, 1.000000000000000000, 0.8660254037844387076, 1.000000000000000000, 0.8660254037844387076, 1.000000000000000000, 0.8660254037844387076, 1.000000000000000000, 0.8660254037844387076, 1.000000000000000000, 0.8660254037844387076, 1.000000000000000000, 0.8660254037844387076, 1.000000000000000000, 0.8660254037844387076, 1.000000000000000000, 0.8660254037844387076, 1.000000000000000000, 0.8660254037844387076, 1.000000000000000000, 0.8660254037844387076, 1.000000000000000000, 0.8660254037844387076, 1.000000000000000000, 0.8660254037844387076, 1.000000000000000000, 0.8660254037844387076, 1.000000000000000000, 0.8660254037844387076, 1.000000000000000000, 0.8660254037844387076, 1.000000000000000000, 0.8660254037844387076, 1.000000000000000000, 0.8660254037844387076, 1.000000000000000000, 0.8660254037844387076, 1.000000000000000000, 0.8660254037844387076, 1.000000000000000000, 0.8660254037844387076, 1.000000000000000000, 0.8660254037844387076, 1.000000000000000000, 0.8660254037844387076, 1.000000000000000000, 0.8660254037844387076, 1.000000000000000000, 0.8660254037844387076, 1.000000000000000000, 0.8660254037844387076, 1.000000000000000000, 0.9111405360107182050, 0.9401542295229976531),
 ( 1.000000000000000000, 0.8660254037844387076, 1.000000000000000000, 0.8660254037844387076, 1.000000000000000000, 0.8660254037844387076, 1.000000000000000000, 0.8660254037844387076, 1.000000000000000000, 0.8660254037844387076, 1.000000000000000000, 0.8660254037844387076, 1.000000000000000000, 0.8660254037844387076, 1.000000000000000000, 0.8660254037844387076, 1.000000000000000000, 0.8660254037844387076, 1.000000000000000000, 0.8660254037844387076, 1.000000000000000000, 0.8660254037844387076, 1.000000000000000000, 0.8660254037844387076, 1.000000000000000000, 0.8660254037844387076, 1.000000000000000000, 0.8660254037844387076, 1.000000000000000000, 0.8660254037844387076, 1.000000000000000000, 0.8660254037844387076, 1.000000000000000000, 0.8660254037844387076, 1.000000000000000000, 0.8660254037844387076, 1.000000000000000000, 0.8660254037844387076, 1.000000000000000000, 0.8660254037844387076, 1.000000000000000000, 0.8660254037844387076, 1.000000000000000000, 0.8660254037844387076, 1.000000000000000000, 0.8660254037844387076, 1.000000000000000000, 0.8660254037844387076, 1.000000000000000000, 0.8660254037844387076, 1.000000000000000000, 0.8660254037844387076, 1.000000000000000000, 0.8660254037844387076, 1.000000000000000000, 0.8660254037844387076, 1.000000000000000000, 0.8660254037844387076, 1.000000000000000000, 0.8660254037844387076, 1.000000000000000000, 0.8660254037844387076, 1.000000000000000000, 0.8660254037844387076, 1.000000000000000000, 0.8660254037844387076, 1.000000000000000000, 0.8660254037844387076, 1.000000000000000000, 0.8660254037844387076, 1.000000000000000000, 0.8660254037844387076, 1.000000000000000000, 0.8660254037844387076, 1.000000000000000000, 0.8660254037844387076, 1.000000000000000000, 0.8660254037844387076, 1.000000000000000000, 0.8660254037844387076, 1.000000000000000000, 0.8660254037844387076, 1.000000000000000000, 0.8660254037844387076, 1.000000000000000000, 0.8660254037844387076, 1.000000000000000000, 0.8660254037844387076, 1.000000000000000000, 0.8660254037844387076, 1.000000000000000000, 0.8660254037844387076, 1.000000000000000000, 0.8660254037844387076, 1.000000000000000000, 0.8660254037844387076, 1.000000000000000000, 0.8660254037844387076, 1.000000000000000000, 0.8660254037844387076, 1.000000000000000000, 0.8660254037844387076, 1.000000000000000000, 0.8660254037844387076, 1.000000000000000000, 0.8660254037844387076, 1.000000000000000000, 0.8660254037844387076, 1.000000000000000000, 0.8660254037844387076, 1.000000000000000000, 0.8660254037844387076, 1.000000000000000000, 0.8660254037844387076, 1.000000000000000000, 0.8660254037844387076, 1.000000000000000000, 0.8660254037844387076, 1.000000000000000000, 0.8660254037844387076, 1.000000000000000000, 0.8660254037844387076, 1.000000000000000000, 0.8660254037844387076, 1.000000000000000000, 0.8660254037844387076, 1.000000000000000000, 0.8660254037844387076, 1.000000000000000000, 0.8660254037844387076, 1.000000000000000000, 0.8660254037844387076, 1.000000000000000000, 0.9111405360107182050, 0.9401542295229976531) ) ) 
 REPRESENTATION_ITEM ( '' )  SURFACE ( )  );
#5242=CARTESIAN_POINT ( 'NONE',  ( -1.595409442497313560E-16, -0.8156249993854829405, -2.605501347177161087 ) ) ;
#5253=AXIS2_PLACEMENT_3D ( 'NONE', #2127, #1400, #2069 ) ;
#5259=CARTESIAN_POINT ( 'NONE',  ( -1.249999999999998224, -4.875000000000000000, 2.165063509461097713 ) ) ;
#5266=CARTESIAN_POINT ( 'NONE',  ( -9.703070624755296135E-15, -3.881249998770965881, 2.500000000000000444 ) ) ;
#5268=LINE ( 'NONE', #3125, #7074 ) ;
#5273=CARTESIAN_POINT ( 'NONE',  ( 2.500000000000000000, -2.474999999999999645, -3.061616997868383141E-16 ) ) ;
#5277=CARTESIAN_POINT ( 'NONE',  ( -2.256430356250000102, -2.053124999385482763, 0.000000000000000000 ) ) ;
#5289=CARTESIAN_POINT ( 'NONE',  ( -1.128215178124998497, -0.5156249993854828961, 1.954126010382872147 ) ) ;
#5290=CARTESIAN_POINT ( 'NONE',  ( -2.500000000000000000, -4.049999999999999822, 0.000000000000000000 ) ) ;
#5293=AXIS2_PLACEMENT_3D ( 'NONE', #2193, #3763, #2248 ) ;
#5300=ADVANCED_FACE ( 'NONE', ( #9924, #4955 ), #8156, .T. ) ;
#5302=CARTESIAN_POINT ( 'NONE',  ( -2.256430356250000102, -2.090624999385482852, -1.302750673588580321 ) ) ;
#5303=EDGE_LOOP ( 'NONE', ( #9930, #1460, #8687, #1583 ) ) ;
#5309=CARTESIAN_POINT ( 'NONE',  ( -1.128215178125000273, -1.228124999385483029, -1.954126010382871259 ) ) ;
#5315=VECTOR ( 'NONE', #1532, 1000.000000000000000 ) ;
#5318=CARTESIAN_POINT ( 'NONE',  ( -0.6698729810778081273, -2.551346188203300169, 2.499999999999999112 ) ) ;
#5319=CARTESIAN_POINT ( 'NONE',  ( 2.500000000000000000, -2.887500000000000178, -1.443375672974065438 ) ) ;
#5322=CARTESIAN_POINT ( 'NONE',  ( -2.500000000000000000, -4.443749998770965881, 0.000000000000000000 ) ) ;
#5323=CARTESIAN_POINT ( 'NONE',  ( -1.128215178125000273, -1.115624999385482985, -1.954126010382871259 ) ) ;
#5324=VECTOR ( 'NONE', #2553, 1000.000000000000000 ) ;
#5326=ORIENTED_EDGE ( 'NONE', *, *, #4474, .F. ) ;
#5328=CARTESIAN_POINT ( 'NONE',  ( -0.6698729810778063509, -0.9361538093386314596, -2.500000000000000000 ) ) ;
#5337=CARTESIAN_POINT ( 'NONE',  ( -1.767625397874844694E-16, -1.462499999999999911, -2.886751345948128655 ) ) ;
#5340=CARTESIAN_POINT ( 'NONE',  ( 2.500000000000000444, -3.862499999999999822, 1.443375672974063439 ) ) ;
#5341=CARTESIAN_POINT ( 'NONE',  ( -1.595409442497313560E-16, -1.715624999385482630, -2.605501347177161087 ) ) ;
#5344=ORIENTED_EDGE ( 'NONE', *, *, #3854, .T. ) ;
#5345=EDGE_LOOP ( 'NONE', ( #8886, #5872, #6019, #1289 ) ) ;
#5351=CARTESIAN_POINT ( 'NONE',  ( 2.256430356249999658, -1.678124999385482541, -1.302750673588581432 ) ) ;
#5359=CARTESIAN_POINT ( 'NONE',  ( 0.6698729810778050187, -2.961153809338631593, 2.500000000000000444 ) ) ;
#5366=CARTESIAN_POINT ( 'NONE',  ( -2.256430356250000102, -1.603124999385482807, 0.000000000000000000 ) ) ;
#5368=CARTESIAN_POINT ( 'NONE',  ( 1.250000000000001110, -0.7499999999999998890, 2.165063509461096380 ) ) ;
#5370=ADVANCED_FACE ( 'NONE', ( #4648 ), #10142, .F. ) ;
#5371=CARTESIAN_POINT ( 'NONE',  ( 1.128215178125001161, -2.353124999385482585, 1.954126010382870815 ) ) ;
#5379=CARTESIAN_POINT ( 'NONE',  ( 2.500000000000000444, -1.162499999999999645, 1.443375672974063439 ) ) ;
#5381=CARTESIAN_POINT ( 'NONE',  ( -2.256430356250000102, -0.6281249993854829405, -1.302750673588580321 ) ) ;
#5386=FACE_OUTER_BOUND ( 'NONE', #3897, .T. ) ;
#5395=CARTESIAN_POINT ( 'NONE',  ( 1.249999999999999334, -3.750000000000000000, -2.165063509461096825 ) ) ;
#5398=CARTESIAN_POINT ( 'NONE',  ( 2.256430356250000546, -1.865624999385482985, 1.302750673588579877 ) ) ;
#5408=CARTESIAN_POINT ( 'NONE',  ( -2.256430356250000102, -0.6281249993854829405, -1.302750673588580321 ) ) ;
#5411=CARTESIAN_POINT ( 'NONE',  ( -2.256430356250000102, -1.490624999385482763, 0.000000000000000000 ) ) ;
#5415=CARTESIAN_POINT ( 'NONE',  ( 2.500000000000000000, -2.831249998770965615, -1.443375672974065438 ) ) ;
#5416=AXIS2_PLACEMENT_3D ( 'NONE', #99, #6528, #935 ) ;
#5424=CARTESIAN_POINT ( 'NONE',  ( -2.256430356250000102, -3.890624999385482674, -1.302750673588580321 ) ) ;
#5429=CARTESIAN_POINT ( 'NONE',  ( -1.595409442497313560E-16, -0.3656249993854829294, -2.605501347177161087 ) ) ;
#5431=FACE_BOUND ( 'NONE', #4503, .T. ) ;
#5433=CARTESIAN_POINT ( 'NONE',  ( -1.250000000000000222, -1.818749998770965881, -2.165063509461096825 ) ) ;
#5438=CARTESIAN_POINT ( 'NONE',  ( 3.061616997868383141E-16, 0.000000000000000000, 2.500000000000000000 ) ) ;
#5439=CARTESIAN_POINT ( 'NONE',  ( -1.128215178124998497, -2.765624999385482674, 1.954126010382872147 ) ) ;
#5444=ORIENTED_EDGE ( 'NONE', *, *, #3465, .T. ) ;
#5447=ORIENTED_EDGE ( 'NONE', *, *, #181, .F. ) ;
#5448=CARTESIAN_POINT ( 'NONE',  ( -0.7756784236033643642, -5.052895385698252362, -2.964907715781667452 ) ) ;
#5449=EDGE_CURVE ( 'NONE', #10235, #4631, #7853, .T. ) ;
#5450=VECTOR ( 'NONE', #5975, 1000.000000000000000 ) ;
#5451=CARTESIAN_POINT ( 'NONE',  ( -8.673617379884035472E-16, -15.00000000000000000, 3.464101615137756163 ) ) ;
#5452=CARTESIAN_POINT ( 'NONE',  ( 4.786228327491941173E-16, -1.040624999385482585, 2.605501347177161087 ) ) ;
#5459=CARTESIAN_POINT ( 'NONE',  ( -1.250000000000000222, -3.168749998770965526, -2.165063509461096825 ) ) ;
#5460=CARTESIAN_POINT ( 'NONE',  ( 9.877377282685029372E-16, -1.181249998770965703, 2.500000000000000000 ) ) ;
#5462=CARTESIAN_POINT ( 'NONE',  ( -2.256430356250000102, -1.528124999385482852, -1.302750673588580321 ) ) ;
#5464=CARTESIAN_POINT ( 'NONE',  ( 2.256430356250000546, -2.653124999385482852, 1.302750673588579877 ) ) ;
#5471=VERTEX_POINT ( 'NONE', #829 ) ;
#5473=DIRECTION ( 'NONE',  ( 0.000000000000000000, 0.000000000000000000, -1.000000000000000000 ) ) ;
#5474=CARTESIAN_POINT ( 'NONE',  ( -1.128215178125000273, -4.378124999385482496, -1.954126010382871259 ) ) ;
#5475=ORIENTED_EDGE ( 'NONE', *, *, #4900, .F. ) ;
#5478=CARTESIAN_POINT ( 'NONE',  ( -3.486133158594716510E-16, -4.106249998770965526, -2.500000000000000000 ) ) ;
#5480=CARTESIAN_POINT ( 'NONE',  ( 1.128215178125001161, -1.003124999385482718, 1.954126010382870815 ) ) ;
#5484=CARTESIAN_POINT ( 'NONE',  ( -2.500000000000000000, -1.837499999999999911, -1.443375672974064106 ) ) ;
#5485=CARTESIAN_POINT ( 'NONE',  ( -1.249999999999998224, -3.018749998770965615, 2.165063509461097713 ) ) ;
#5490=CARTESIAN_POINT ( 'NONE',  ( -2.256430356250000102, -1.978124999385482807, -1.302750673588580321 ) ) ;
#5501=CARTESIAN_POINT ( 'NONE',  ( -2.499999999999999556, -4.012499999999999289, 1.443375672974065882 ) ) ;
#5503=EDGE_CURVE ( 'NONE', #5726, #6080, #7102, .T. ) ;
#5506=CARTESIAN_POINT ( 'NONE',  ( 4.786228327491941173E-16, -4.190624999385482496, 2.605501347177161087 ) ) ;
#5513=CARTESIAN_POINT ( 'NONE',  ( 1.128215178124999607, -2.990624999385482763, -1.954126010382871259 ) ) ;
#5516=CARTESIAN_POINT ( 'NONE',  ( 1.128215178124999607, -2.990624999385482763, -1.954126010382871259 ) ) ;
#5524=VERTEX_POINT ( 'NONE', #9520 ) ;
#5525=CARTESIAN_POINT ( 'NONE',  ( 2.256430356250000546, -5.015624999385482674, 1.302750673588579877 ) ) ;
#5531=CARTESIAN_POINT ( 'NONE',  ( -2.256430356249998770, -2.465624999385482852, 1.302750673588581876 ) ) ;
#5534=DIRECTION ( 'NONE',  ( 0.000000000000000000, -1.000000000000000000, 0.000000000000000000 ) ) ;
#5536=CARTESIAN_POINT ( 'NONE',  ( -1.250000000000000222, -2.268749998770965615, -2.165063509461096825 ) ) ;
#5541=CARTESIAN_POINT ( 'NONE',  ( -1.128215178125000273, -4.715624999385481964, -1.954126010382871259 ) ) ;
#5542=ORIENTED_EDGE ( 'NONE', *, *, #2183, .F. ) ;
#5545=CARTESIAN_POINT ( 'NONE',  ( -0.6698729810778054627, -3.451346188203299192, 2.500000000000000000 ) ) ;
#5549=CARTESIAN_POINT ( 'NONE',  ( 2.500000000000000000, -3.374999999999999556, -3.061616997868383141E-16 ) ) ;
#5551=CARTESIAN_POINT ( 'NONE',  ( -2.256430356250000102, -4.340624999385482852, -1.302750673588580321 ) ) ;
#5559=CARTESIAN_POINT ( 'NONE',  ( 1.128215178124999607, -2.540624999385482585, -1.954126010382871259 ) ) ;
#5562=CARTESIAN_POINT ( 'NONE',  ( -2.256430356250000102, -1.528124999385482630, -1.302750673588580321 ) ) ;
#5565=DIRECTION ( 'NONE',  ( 0.000000000000000000, -1.000000000000000000, 0.000000000000000000 ) ) ;
#5571=CARTESIAN_POINT ( 'NONE',  ( -2.500000000000000000, 0.000000000000000000, 0.000000000000000000 ) ) ;
#5574=CARTESIAN_POINT ( 'NONE',  ( -1.728532663107115397, -5.253648270121824559, -1.450397457657151001 ) ) ;
#5580=CARTESIAN_POINT ( 'NONE',  ( 2.256430356249999658, -2.690624999385482941, -1.302750673588581432 ) ) ;
#5585=AXIS2_PLACEMENT_3D ( 'NONE', #2781, #2154, #10111 ) ;
#5587=CARTESIAN_POINT ( 'NONE',  ( -2.500000000000000000, -1.331249998770965615, -1.443375672974064106 ) ) ;
#5588=ORIENTED_EDGE ( 'NONE', *, *, #10255, .T. ) ;
#5592=CARTESIAN_POINT ( 'NONE',  ( 4.786228327491941173E-16, -4.078124999385482674, 2.605501347177161087 ) ) ;
#5594=DIRECTION ( 'NONE',  ( 0.000000000000000000, 0.9949358851208914833, -0.1005116137503925394 ) ) ;
#5598=EDGE_LOOP ( 'NONE', ( #6608, #2156, #4161, #8077 ) ) ;
#5599=CARTESIAN_POINT ( 'NONE',  ( 1.250000000000001110, -3.899999999999999911, 2.165063509461096380 ) ) ;
#5600=VECTOR ( 'NONE', #7228, 1000.000000000000000 ) ;
#5602=CARTESIAN_POINT ( 'NONE',  ( 4.786228327491941173E-16, -5.090624999385482852, 2.605501347177161087 ) ) ;
#5610=CARTESIAN_POINT ( 'NONE',  ( 4.786228327491940187E-16, -4.528124999385482852, 2.605501347177161087 ) ) ;
#5612=AXIS2_PLACEMENT_3D ( 'NONE', #2614, #5855, #2770 ) ;
#5614=CARTESIAN_POINT ( 'NONE',  ( -1.128215178125000273, -2.915624999385482585, -1.954126010382871259 ) ) ;
#5617=EDGE_CURVE ( 'NONE', #3111, #1260, #4799, .T. ) ;
#5624=CARTESIAN_POINT ( 'NONE',  ( 1.128215178125001161, -4.603124999385482141, 1.954126010382870815 ) ) ;
#5628=CARTESIAN_POINT ( 'NONE',  ( 2.256430356250000102, -4.978124999385482141, -2.763330213280484622E-16 ) ) ;
#5634=CARTESIAN_POINT ( 'NONE',  ( 5.302876193624534821E-16, -1.631249998770965881, 2.886751345948128655 ) ) ;
#5637=LINE ( 'NONE', #7302, #4791 ) ;
#5640=CARTESIAN_POINT ( 'NONE',  ( -1.128215178124998497, -3.665624999385482585, 1.954126010382872147 ) ) ;
#5643=ORIENTED_EDGE ( 'NONE', *, *, #1450, .T. ) ;
#5648=CARTESIAN_POINT ( 'NONE',  ( 0.000000000000000000, -20.00000000000000000, -2.500000000000000444 ) ) ;
#5652=EDGE_CURVE ( 'NONE', #9254, #2231, #2721, .T. ) ;
#5654=CARTESIAN_POINT ( 'NONE',  ( 4.786228327491941173E-16, -4.640624999385482674, 2.605501347177161087 ) ) ;
#5656=( BOUNDED_CURVE ( )  B_SPLINE_CURVE ( 2, ( #159, #7466, #1141, #3440, #6582, #990, #2612, #9773, #9151 ),
 .UNSPECIFIED., .F., .F. ) 
 B_SPLINE_CURVE_WITH_KNOTS ( ( 3, 2, 2, 2, 3 ),
 ( 0.8541666666666667407, 0.8611111111111111605, 0.8750000000000000000, 0.8888888888888888395, 0.8958333333333333703 ),
 .UNSPECIFIED. ) 
 CURVE ( )  GEOMETRIC_REPRESENTATION_ITEM ( )  RATIONAL_B_SPLINE_CURVE ( ( 0.9330127018922192983, 0.9330127018922198534, 1.000000000000000000, 0.8660254037844387076, 1.000000000000000000, 0.8660254037844387076, 1.000000000000000000, 0.9330127018922187432, 0.9330127018922192983 ) ) 
 REPRESENTATION_ITEM ( '' )  );
#5661=CARTESIAN_POINT ( 'NONE',  ( 9.877377282685029372E-16, -4.781249998770965348, 2.500000000000000000 ) ) ;
#5663=CARTESIAN_POINT ( 'NONE',  ( 2.256430356250000546, -3.103124999385482585, 1.302750673588579877 ) ) ;
#5665=EDGE_LOOP ( 'NONE', ( #9298, #7365, #8162, #4184 ) ) ;
#5666=CARTESIAN_POINT ( 'NONE',  ( -2.256430356250000102, -4.228124999385483029, -1.302750673588580321 ) ) ;
#5671=VECTOR ( 'NONE', #5040, 1000.000000000000000 ) ;
#5676=CARTESIAN_POINT ( 'NONE',  ( 2.500000000000000444, -5.156249998770965348, 1.443375672974063439 ) ) ;
#5681=CARTESIAN_POINT ( 'NONE',  ( -2.256430356250000102, -3.440624999385482496, -1.302750673588580321 ) ) ;
#5686=CARTESIAN_POINT ( 'NONE',  ( -1.249999999999998224, -4.818749998770964993, 2.165063509461097713 ) ) ;
#5690=CARTESIAN_POINT ( 'NONE',  ( -1.250000000000000222, -3.224999999999999645, -2.165063509461096825 ) ) ;
#5692=CARTESIAN_POINT ( 'NONE',  ( -1.128215178125000273, -3.365624999385482763, -1.954126010382871259 ) ) ;
#5695=ORIENTED_EDGE ( 'NONE', *, *, #8350, .F. ) ;
#5697=CARTESIAN_POINT ( 'NONE',  ( -8.673617379884035472E-16, -15.00000000000000000, 3.464101615137756163 ) ) ;
#5698=DIRECTION ( 'NONE',  ( 0.000000000000000000, 0.9961946980917455452, -0.08715574274765836016 ) ) ;
#5703=CARTESIAN_POINT ( 'NONE',  ( 1.128215178125001161, -3.253124999385482496, 1.954126010382870815 ) ) ;
#5707=ADVANCED_FACE ( 'NONE', ( #8123 ), #4241, .T. ) ;
#5713=CARTESIAN_POINT ( 'NONE',  ( -2.256430356249998770, -3.703124999385482674, 1.302750673588581876 ) ) ;
#5715=ORIENTED_EDGE ( 'NONE', *, *, #9765, .F. ) ;
#5716=CARTESIAN_POINT ( 'NONE',  ( -2.256430356249999214, -4.603124999385482141, 1.302750673588581876 ) ) ;
#5722=VERTEX_POINT ( 'NONE', #166 ) ;
#5723=CARTESIAN_POINT ( 'NONE',  ( 2.500000000000000000, -3.374999999999999556, -3.061616997868383141E-16 ) ) ;
#5725=ORIENTED_EDGE ( 'NONE', *, *, #7478, .T. ) ;
#5726=VERTEX_POINT ( 'NONE', #3558 ) ;
#5728=CARTESIAN_POINT ( 'NONE',  ( 0.6698729810778025762, -4.311153809338631682, 2.500000000000002665 ) ) ;
#5731=CARTESIAN_POINT ( 'NONE',  ( 4.786228327491940187E-16, -3.290624999385482585, 2.605501347177161087 ) ) ;
#5734=CARTESIAN_POINT ( 'NONE',  ( 2.500000000000000000, -5.118749998770964815, -3.061616997868383141E-16 ) ) ;
#5737=DIRECTION ( 'NONE',  ( 0.8660254037844384856, 0.000000000000000000, 0.5000000000000003331 ) ) ;
#5739=CARTESIAN_POINT ( 'NONE',  ( -2.256430356249999214, -4.153124999385482852, 1.302750673588581876 ) ) ;
#5740=B_SPLINE_CURVE_WITH_KNOTS ( 'NONE', 1,
 ( #806, #5571 ),
 .UNSPECIFIED., .F., .F.,
 ( 2, 2 ),
 ( 0.000000000000000000, 1.000000000000000000 ),
 .UNSPECIFIED. ) ;
#5743=CARTESIAN_POINT ( 'NONE',  ( 1.250000000000001110, -1.649999999999999689, 2.165063509461096380 ) ) ;
#5750=DIRECTION ( 'NONE',  ( -0.000000000000000000, -1.000000000000000000, -0.000000000000000000 ) ) ;
#5758=EDGE_CURVE ( 'NONE', #2494, #4882, #8922, .T. ) ;
#5760=ORIENTED_EDGE ( 'NONE', *, *, #4556, .F. ) ;
#5761=CARTESIAN_POINT ( 'NONE',  ( 2.256430356249999658, -4.828124999385483562, -1.302750673588581432 ) ) ;
#5762=EDGE_CURVE ( 'NONE', #5524, #2954, #9981, .T. ) ;
#5764=CARTESIAN_POINT ( 'NONE',  ( -2.256430356250000102, -0.7031249993854828961, 0.000000000000000000 ) ) ;
#5774=CARTESIAN_POINT ( 'NONE',  ( -2.256430356249998770, -2.915624999385482585, 1.302750673588581876 ) ) ;
#5776=CIRCLE ( 'NONE', #929, 0.4999999999999953371 ) ;
#5777=CARTESIAN_POINT ( 'NONE',  ( -1.250000000000000222, -1.875000000000000000, -2.165063509461096825 ) ) ;
#5778=CARTESIAN_POINT ( 'NONE',  ( -1.915118561403101882, -5.394273269507308122, -1.606960141313192425 ) ) ;
#5779=EDGE_LOOP ( 'NONE', ( #3538, #3471, #5588, #4642 ) ) ;
#5784=CARTESIAN_POINT ( 'NONE',  ( 1.249999999999999334, -1.499999999999999778, -2.165063509461096825 ) ) ;
#5806=ORIENTED_EDGE ( 'NONE', *, *, #8836, .F. ) ;
#5807=CARTESIAN_POINT ( 'NONE',  ( 1.128215178124999607, -4.340624999385482852, -1.954126010382871259 ) ) ;
#5808=FILL_AREA_STYLE_COLOUR ( '', #4139 ) ;
#5809=CARTESIAN_POINT ( 'NONE',  ( -1.249999999999998224, -2.624999999999999556, 2.165063509461097713 ) ) ;
#5814=AXIS2_PLACEMENT_3D ( 'NONE', #10086, #9297, #8409 ) ;
#5824=DIRECTION ( 'NONE',  ( 0.000000000000000000, -1.000000000000000000, 0.000000000000000000 ) ) ;
#5827=CARTESIAN_POINT ( 'NONE',  ( 5.302876193624534821E-16, -5.231249998770965526, 2.886751345948128655 ) ) ;
#5829=EDGE_CURVE ( 'NONE', #6080, #3756, #1754, .T. ) ;
#5840=CARTESIAN_POINT ( 'NONE',  ( 4.996790860652426159E-15, -2.306249998770965259, -2.500000000000000000 ) ) ;
#5845=CARTESIAN_POINT ( 'NONE',  ( 1.045839947578414805E-15, -0.5625000000000001110, -2.500000000000000000 ) ) ;
#5850=CARTESIAN_POINT ( 'NONE',  ( -1.250000000000000222, -0.07499999999999999722, -2.165063509461096825 ) ) ;
#5851=VERTEX_POINT ( 'NONE', #3249 ) ;
#5853=CARTESIAN_POINT ( 'NONE',  ( -2.256430356250000102, -4.190624999385482496, 0.000000000000000000 ) ) ;
#5855=DIRECTION ( 'NONE',  ( 0.000000000000000000, -1.000000000000000000, 0.000000000000000000 ) ) ;
#5867=CARTESIAN_POINT ( 'NONE',  ( -2.499999999999999112, -1.706249998770965615, 1.443375672974065882 ) ) ;
#5870=ADVANCED_BREP_SHAPE_REPRESENTATION ( '', ( #2806, #5055 ), #7312 ) ;
#5872=ORIENTED_EDGE ( 'NONE', *, *, #6253, .F. ) ;
#5874=AXIS2_PLACEMENT_3D ( 'NONE', #1502, #2975, #6370 ) ;
#5875=CARTESIAN_POINT ( 'NONE',  ( 1.250000000000001110, -3.843749998770965348, 2.165063509461096380 ) ) ;
#5887=DIRECTION ( 'NONE',  ( 0.000000000000000000, -1.000000000000000000, 0.000000000000000000 ) ) ;
#5888=CARTESIAN_POINT ( 'NONE',  ( 2.500000000000000444, -2.512500000000000178, 1.443375672974063439 ) ) ;
#5902=CARTESIAN_POINT ( 'NONE',  ( -1.728530063377412107, -5.141148402510967053, -1.450400555903694988 ) ) ;
#5903=CARTESIAN_POINT ( 'NONE',  ( 2.500000000000000000, -0.6749999999999999334, -3.061616997868383141E-16 ) ) ;
#5907=CARTESIAN_POINT ( 'NONE',  ( -3.486133158594716510E-16, -1.012499999999999956, -2.500000000000000000 ) ) ;
#5908=DIRECTION ( 'NONE',  ( 0.000000000000000000, -1.000000000000000000, 0.000000000000000000 ) ) ;
#5911=EDGE_LOOP ( 'NONE', ( #10260, #57, #1439, #6444 ) ) ;
#5912=( BOUNDED_CURVE ( )  B_SPLINE_CURVE ( 2, ( #10134, #5318, #3695, #10018, #10195, #2853, #10073, #1337, #2802 ),
 .UNSPECIFIED., .F., .T. ) 
 B_SPLINE_CURVE_WITH_KNOTS ( ( 3, 2, 2, 2, 3 ),
 ( 0.3958333333333333703, 0.4027777777777777901, 0.4166666666666666852, 0.4305555555555555802, 0.4375000000000000000 ),
 .UNSPECIFIED. ) 
 CURVE ( )  GEOMETRIC_REPRESENTATION_ITEM ( )  RATIONAL_B_SPLINE_CURVE ( ( 0.9330127018922194093, 0.9330127018922196314, 1.000000000000000000, 0.8660254037844387076, 1.000000000000000000, 0.8660254037844387076, 1.000000000000000000, 0.9330127018922194093, 0.9330127018922194093 ) ) 
 REPRESENTATION_ITEM ( '' )  );
#5914=CARTESIAN_POINT ( 'NONE',  ( 0.000000000000000000, -15.00000000000000000, -2.500000000000000000 ) ) ;
#5915=FACE_OUTER_BOUND ( 'NONE', #1339, .T. ) ;
#5923=CARTESIAN_POINT ( 'NONE',  ( 1.128215178125001161, -2.353124999385482585, 1.954126010382870815 ) ) ;
#5937=CARTESIAN_POINT ( 'NONE',  ( 2.500000000000000000, -0.6187499987709659255, -3.061616997868383141E-16 ) ) ;
#5938=ADVANCED_FACE ( 'NONE', ( #8111 ), #6675, .T. ) ;
#5954=FACE_OUTER_BOUND ( 'NONE', #7501, .T. ) ;
#5955=VERTEX_POINT ( 'NONE', #5104 ) ;
#5957=CARTESIAN_POINT ( 'NONE',  ( -1.250000000000000222, -4.968749998770965348, -2.165063509461096825 ) ) ;
#5958=ORIENTED_EDGE ( 'NONE', *, *, #172, .T. ) ;
#5961=CARTESIAN_POINT ( 'NONE',  ( 5.302876193624534821E-16, -0.7874999999999998668, 2.886751345948128655 ) ) ;
#5965=AXIS2_PLACEMENT_3D ( 'NONE', #3108, #4872, #742 ) ;
#5966=CARTESIAN_POINT ( 'NONE',  ( 9.877377282685029372E-16, -1.237499999999999600, 2.500000000000000000 ) ) ;
#5971=CARTESIAN_POINT ( 'NONE',  ( -1.128215178125000273, -0.6656249993854829183, -1.954126010382871259 ) ) ;
#5972=CARTESIAN_POINT ( 'NONE',  ( -2.256430356250000102, -0.1406249993854829794, 0.000000000000000000 ) ) ;
#5975=DIRECTION ( 'NONE',  ( 0.000000000000000000, -1.000000000000000000, 0.000000000000000000 ) ) ;
#5979=CARTESIAN_POINT ( 'NONE',  ( 4.786228327491941173E-16, -1.490624999385482985, 2.605501347177161087 ) ) ;
#5985=EDGE_CURVE ( 'NONE', #10235, #4027, #4228, .T. ) ;
#5988=CARTESIAN_POINT ( 'NONE',  ( 2.500000000000000000, -2.474999999999999645, -3.061616997868383141E-16 ) ) ;
#5991=CARTESIAN_POINT ( 'NONE',  ( -3.486133158594716510E-16, -2.756249998770965437, -2.500000000000000000 ) ) ;
#5998=DIRECTION ( 'NONE',  ( 0.000000000000000000, -1.000000000000000000, 0.000000000000000000 ) ) ;
#6005=CARTESIAN_POINT ( 'NONE',  ( 2.500000000000000444, -2.062499999999999556, 1.443375672974063439 ) ) ;
#6007=CARTESIAN_POINT ( 'NONE',  ( -1.128215178124998497, -2.428124999385482763, 1.954126010382872147 ) ) ;
#6008=ADVANCED_FACE ( 'NONE', ( #986 ), #9769, .T. ) ;
#6014=CARTESIAN_POINT ( 'NONE',  ( -4.357666448243394824E-15, -2.981249998770965526, 2.500000000000000000 ) ) ;
#6017=CARTESIAN_POINT ( 'NONE',  ( -2.256430356249998770, -1.003124999385482718, 1.302750673588581876 ) ) ;
#6019=ORIENTED_EDGE ( 'NONE', *, *, #4805, .F. ) ;
#6020=CARTESIAN_POINT ( 'NONE',  ( 2.256430356250000546, -0.8531249993854828073, 1.302750673588579877 ) ) ;
#6027=ORIENTED_EDGE ( 'NONE', *, *, #843, .F. ) ;
#6028=DIRECTION ( 'NONE',  ( -0.04357787137382922171, -0.9961946980917455452, 0.07547908730517349785 ) ) ;
#6029=CARTESIAN_POINT ( 'NONE',  ( 2.256430356250000546, -2.765624999385483118, 1.302750673588579877 ) ) ;
#6030=ORIENTED_EDGE ( 'NONE', *, *, #4456, .F. ) ;
#6035=VERTEX_POINT ( 'NONE', #5845 ) ;
#6037=CARTESIAN_POINT ( 'NONE',  ( -2.500000000000000000, -0.8812499987709659921, -1.443375672974064106 ) ) ;
#6039=CARTESIAN_POINT ( 'NONE',  ( 0.6698729810778075722, -3.017403810567666156, 2.499999999999999556 ) ) ;
#6048=CARTESIAN_POINT ( 'NONE',  ( -1.249999999999998224, -3.918749998770965082, 2.165063509461097713 ) ) ;
#6050=CARTESIAN_POINT ( 'NONE',  ( -0.6698729810778063509, -0.5424038105676658450, -2.500000000000000000 ) ) ;
#6055=CARTESIAN_POINT ( 'NONE',  ( 2.500000000000000000, -2.024999999999999911, -3.061616997868383141E-16 ) ) ;
#6059=CARTESIAN_POINT ( 'NONE',  ( 1.128215178124999607, -2.203124999385482674, -1.954126010382871259 ) ) ;
#6066=CARTESIAN_POINT ( 'NONE',  ( 1.034219503716432668E-14, -3.206249998770966059, -2.500000000000000000 ) ) ;
#6070=CARTESIAN_POINT ( 'NONE',  ( -2.256430356249998770, -0.5531249993854828739, 1.302750673588581876 ) ) ;
#6071=CARTESIAN_POINT ( 'NONE',  ( -9.703070624755296135E-15, -5.231249998770965526, 2.500000000000000444 ) ) ;
#6073=CARTESIAN_POINT ( 'NONE',  ( -2.500000000000000000, -1.293749998770965970, 0.000000000000000000 ) ) ;
#6080=VERTEX_POINT ( 'NONE', #8578 ) ;
#6082=EDGE_CURVE ( 'NONE', #6810, #4141, #10085, .T. ) ;
#6084=CARTESIAN_POINT ( 'NONE',  ( -2.256430356250000102, -2.503124999385482496, 0.000000000000000000 ) ) ;
#6087=CARTESIAN_POINT ( 'NONE',  ( 2.500000000000000444, -0.7124999999999999112, 1.443375672974063439 ) ) ;
#6088=CARTESIAN_POINT ( 'NONE',  ( 1.249999999999999334, -0.1499999999999999944, -2.165063509461096825 ) ) ;
#6089=CARTESIAN_POINT ( 'NONE',  ( 2.256430356250000102, -2.278124999385482852, -2.763330213280484622E-16 ) ) ;
#6098=CARTESIAN_POINT ( 'NONE',  ( -2.256430356250000102, -1.490624999385482763, 0.000000000000000000 ) ) ;
#6104=CARTESIAN_POINT ( 'NONE',  ( -2.499999999999999112, -3.956249998770965615, 1.443375672974065882 ) ) ;
#6106=EDGE_CURVE ( 'NONE', #1163, #1380, #6928, .T. ) ;
#6110=ORIENTED_EDGE ( 'NONE', *, *, #7485, .T. ) ;
#6111=CARTESIAN_POINT ( 'NONE',  ( -1.249999999999998224, -2.624999999999999556, 2.165063509461097713 ) ) ;
#6114=DIRECTION ( 'NONE',  ( 0.000000000000000000, 0.000000000000000000, -1.000000000000000000 ) ) ;
#6115=CARTESIAN_POINT ( 'NONE',  ( -1.128215178124998497, -2.878124999385482496, 1.954126010382872147 ) ) ;
#6123=VECTOR ( 'NONE', #4465, 1000.000000000000114 ) ;
#6125=CARTESIAN_POINT ( 'NONE',  ( 2.256430356249999658, -2.128124999385482496, -1.302750673588581432 ) ) ;
#6128=CARTESIAN_POINT ( 'NONE',  ( 9.877377282685029372E-16, -1.631249998770965659, 2.500000000000000000 ) ) ;
#6136=VERTEX_POINT ( 'NONE', #9296 ) ;
#6139=CARTESIAN_POINT ( 'NONE',  ( 2.256430356250000546, -1.415624999385482807, 1.302750673588579877 ) ) ;
#6141=CARTESIAN_POINT ( 'NONE',  ( -3.000000000000000888, -15.00000000000000000, 1.732050807568878303 ) ) ;
#6145=CARTESIAN_POINT ( 'NONE',  ( -1.595409442497313560E-16, -2.165624999385483029, -2.605501347177161087 ) ) ;
#6152=CARTESIAN_POINT ( 'NONE',  ( 1.034219503716432668E-14, -2.812500000000000444, -2.500000000000000000 ) ) ;
#6154=CARTESIAN_POINT ( 'NONE',  ( 0.000000000000000000, 0.000000000000000000, -2.500000000000000000 ) ) ;
#6155=CARTESIAN_POINT ( 'NONE',  ( 1.034219503716432668E-14, -4.556249998770965703, -2.500000000000000000 ) ) ;
#6156=CARTESIAN_POINT ( 'NONE',  ( 2.256430356250000546, -2.653124999385482852, 1.302750673588579877 ) ) ;
#6159=EDGE_LOOP ( 'NONE', ( #4945, #4004, #10207, #10117 ) ) ;
#6168=CARTESIAN_POINT ( 'NONE',  ( -2.500000000000000000, -3.600000000000000089, 0.000000000000000000 ) ) ;
#6170=CARTESIAN_POINT ( 'NONE',  ( 2.500000000000000000, -3.787499999999999645, -1.443375672974065438 ) ) ;
#6171=CARTESIAN_POINT ( 'NONE',  ( -1.128215178125000273, -3.028124999385482408, -1.954126010382871259 ) ) ;
#6180=CARTESIAN_POINT ( 'NONE',  ( -1.128215178125000273, -1.115624999385482985, -1.954126010382871259 ) ) ;
#6182=CARTESIAN_POINT ( 'NONE',  ( 2.256430356250000546, -0.4031249993854829627, 1.302750673588579877 ) ) ;
#6187=ADVANCED_FACE ( 'NONE', ( #5386 ), #2186, .T. ) ;
#6193=ORIENTED_EDGE ( 'NONE', *, *, #3622, .F. ) ;
#6194=CARTESIAN_POINT ( 'NONE',  ( 4.786228327491941173E-16, -3.290624999385482585, 2.605501347177161087 ) ) ;
#6199=AXIS2_PLACEMENT_3D ( 'NONE', #7616, #6944, #2762 ) ;
#6200=CARTESIAN_POINT ( 'NONE',  ( -2.256430356250000102, -2.053124999385482763, 0.000000000000000000 ) ) ;
#6204=CARTESIAN_POINT ( 'NONE',  ( 5.302876193624534821E-16, -2.981249998770965970, 2.886751345948128655 ) ) ;
#6210=CARTESIAN_POINT ( 'NONE',  ( -1.128215178124998497, -2.315624999385482941, 1.954126010382872147 ) ) ;
#6214=CARTESIAN_POINT ( 'NONE',  ( -2.499999999999999112, -0.8062499987709659255, 1.443375672974065882 ) ) ;
#6222=ORIENTED_EDGE ( 'NONE', *, *, #1549, .T. ) ;
#6223=CARTESIAN_POINT ( 'NONE',  ( -2.500000000000000000, -4.973640350848739011, -0.9099175284171376887 ) ) ;
#6225=CARTESIAN_POINT ( 'NONE',  ( -2.256430356249999214, -1.115624999385482763, 1.302750673588581876 ) ) ;
#6234=CARTESIAN_POINT ( 'NONE',  ( -1.595409442497313560E-16, -1.153124999385482852, -2.605501347177161087 ) ) ;
#6237=CARTESIAN_POINT ( 'NONE',  ( -1.128215178124998497, -1.415624999385482807, 1.954126010382872147 ) ) ;
#6239=VECTOR ( 'NONE', #7362, 1000.000000000000000 ) ;
#6242=CARTESIAN_POINT ( 'NONE',  ( 2.500000000000000444, -2.906249998770965792, 1.443375672974063439 ) ) ;
#6250=CARTESIAN_POINT ( 'NONE',  ( 1.128215178124999607, -4.003124999385482496, -1.954126010382871259 ) ) ;
#6253=EDGE_CURVE ( 'NONE', #5722, #7541, #5158, .T. ) ;
#6256=CARTESIAN_POINT ( 'NONE',  ( -2.256430356250000102, -2.090624999385482852, -1.302750673588580321 ) ) ;
#6261=CARTESIAN_POINT ( 'NONE',  ( 2.500000000000000444, -2.906249998770965792, 1.443375672974063439 ) ) ;
#6265=( BOUNDED_SURFACE ( )  B_SPLINE_SURFACE ( 1, 2, ( 
 ( #2038, #4507, #10170, #3623, #3007, #7700, #372, #6182, #8327, #4347, #6750, #7530, #3564, #10002, #5971, #9164, #4453, #8379, #425, #6020, #5232, #8432, #1264, #693, #7225, #10329, #1478, #7020, #4041, #7810, #7967, #10224, #9585, #7178, #6237, #7913, #5411, #5562, #4673, #3056, #3258, #4771, #8655, #9439, #4824, #8020, #6394, #747, #60, #7863, #3885, #9636, #10279, #3113, #6447, #801, #8604, #8708, #2316, #3993, #8753, #2266, #7072, #9492, #6294, #7, #852, #5464, #1427, #2417, #6346, #3210, #640, #4616, #5614, #3836, #5516, #1527, #4721, #3940, #8802, #7125, #3162, #9541, #1577, #2365, #1632, #948, #2662, #4235, #7323, #8209, #7367, #8067, #114, #4185, #3305, #8949, #9685, #1728, #5012, #7276, #2568, #208, #4142, #6495, #992, #161, #5853, #5666, #3394, #3349, #5807, #9047, #8163, #899, #4284, #2524, #1041, #5716, #6541, #4876, #5061, #7416, #8262, #5761, #9729, #1768, #4090, #1817, #8903, #6585, #4921, #256, #4963, #8117, #9776 ),
 ( #2613, #8855, #8998, #3443, #1866, #1092, #6634, #9830, #7467, #309, #3497, #6683, #2472, #1683, #9304, #3661, #5113, #6894, #5903, #6789, #1247, #5961, #6841, #2715, #8472, #410, #2768, #7625, #10036, #1143, #2136, #9153, #3605, #1969, #465, #5165, #8311, #10091, #8364, #5337, #1195, #2928, #4437, #7572, #4386, #3549, #6737, #7518, #1299, #1353, #2873, #8528, #9989, #2824, #6055, #6005, #9935, #9198, #2020, #7682, #571, #2079, #9246, #5217, #8416, #4543, #5273, #4490, #520, #4334, #6111, #3711, #7738, #9099, #3765, #9876, #1919, #359, #10155, #1409, #10311, #2988, #9423, #10208, #3097, #8587, #2351, #8741, #9476, #4755, #5549, #1464, #3977, #9366, #10162, #9572, #6168, #7112, #2405, #2195, #5395, #6280, #1513, #4707, #5599, #7057, #2304, #5501, #8004, #7163, #4601, #3196, #3043, #733, #7899, #9526, #6378, #8789, #7793, #3147, #1614, #625, #3823, #8692, #3925, #6332, #4809, #10265, #1564, #7953, #835, #6952, #7004, #6223, #2250, #785, #5448 ) ),
 .UNSPECIFIED., .F., .F., .F. ) 
 B_SPLINE_SURFACE_WITH_KNOTS ( ( 2, 2 ),
 ( 3, 2, 2, 2, 2, 2, 2, 2, 2, 2, 2, 2, 2, 2, 2, 2, 2, 2, 2, 2, 2, 2, 2, 2, 2, 2, 2, 2, 2, 2, 2, 2, 2, 2, 2, 2, 2, 2, 2, 2, 2, 2, 2, 2, 2, 2, 2, 2, 2, 2, 2, 2, 2, 2, 2, 2, 2, 2, 2, 2, 2, 2, 2, 2, 2, 2, 2, 2, 3 ),
 ( 0.000000000000000000, 1.000000000000000000 ),
 ( 0.000000000000000000, 0.01388888888888888812, 0.02777777777777777624, 0.04166666666666666435, 0.05555555555555555247, 0.06944444444444444753, 0.08333333333333332871, 0.09722222222222222376, 0.1111111111111111049, 0.1250000000000000000, 0.1388888888888888951, 0.1527777777777777901, 0.1666666666666666574, 0.1805555555555555525, 0.1944444444444444475, 0.2083333333333333426, 0.2222222222222222099, 0.2361111111111111049, 0.2500000000000000000, 0.2638888888888888951, 0.2777777777777777901, 0.2916666666666666852, 0.3055555555555555802, 0.3194444444444444198, 0.3333333333333333148, 0.3472222222222222099, 0.3611111111111111049, 0.3750000000000000000, 0.3888888888888888951, 0.4027777777777777901, 0.4166666666666666852, 0.4305555555555555802, 0.4444444444444444198, 0.4583333333333333148, 0.4722222222222222099, 0.4861111111111111049, 0.5000000000000000000, 0.5138888888888888395, 0.5277777777777777901, 0.5416666666666666297, 0.5555555555555555802, 0.5694444444444444198, 0.5833333333333333703, 0.5972222222222222099, 0.6111111111111111605, 0.6250000000000000000, 0.6388888888888888395, 0.6527777777777777901, 0.6666666666666666297, 0.6805555555555555802, 0.6944444444444444198, 0.7083333333333333703, 0.7222222222222222099, 0.7361111111111111605, 0.7500000000000000000, 0.7638888888888888395, 0.7777777777777777901, 0.7916666666666666297, 0.8055555555555555802, 0.8194444444444444198, 0.8333333333333333703, 0.8472222222222222099, 0.8611111111111111605, 0.8750000000000000000, 0.8888888888888888395, 0.9027777777777777901, 0.9166666666666666297, 0.9258784821878333071, 0.9351372670097116702 ),
 .UNSPECIFIED. ) 
 GEOMETRIC_REPRESENTATION_ITEM ( )  RATIONAL_B_SPLINE_SURFACE ( (
 ( 1.000000000000000000, 0.8660254037844387076, 1.000000000000000000, 0.8660254037844387076, 1.000000000000000000, 0.8660254037844387076, 1.000000000000000000, 0.8660254037844387076, 1.000000000000000000, 0.8660254037844387076, 1.000000000000000000, 0.8660254037844387076, 1.000000000000000000, 0.8660254037844387076, 1.000000000000000000, 0.8660254037844387076, 1.000000000000000000, 0.8660254037844387076, 1.000000000000000000, 0.8660254037844387076, 1.000000000000000000, 0.8660254037844387076, 1.000000000000000000, 0.8660254037844387076, 1.000000000000000000, 0.8660254037844387076, 1.000000000000000000, 0.8660254037844387076, 1.000000000000000000, 0.8660254037844387076, 1.000000000000000000, 0.8660254037844387076, 1.000000000000000000, 0.8660254037844387076, 1.000000000000000000, 0.8660254037844387076, 1.000000000000000000, 0.8660254037844387076, 1.000000000000000000, 0.8660254037844387076, 1.000000000000000000, 0.8660254037844387076, 1.000000000000000000, 0.8660254037844387076, 1.000000000000000000, 0.8660254037844387076, 1.000000000000000000, 0.8660254037844387076, 1.000000000000000000, 0.8660254037844387076, 1.000000000000000000, 0.8660254037844387076, 1.000000000000000000, 0.8660254037844387076, 1.000000000000000000, 0.8660254037844387076, 1.000000000000000000, 0.8660254037844387076, 1.000000000000000000, 0.8660254037844387076, 1.000000000000000000, 0.8660254037844387076, 1.000000000000000000, 0.8660254037844387076, 1.000000000000000000, 0.8660254037844387076, 1.000000000000000000, 0.8660254037844387076, 1.000000000000000000, 0.8660254037844387076, 1.000000000000000000, 0.8660254037844387076, 1.000000000000000000, 0.8660254037844387076, 1.000000000000000000, 0.8660254037844387076, 1.000000000000000000, 0.8660254037844387076, 1.000000000000000000, 0.8660254037844387076, 1.000000000000000000, 0.8660254037844387076, 1.000000000000000000, 0.8660254037844387076, 1.000000000000000000, 0.8660254037844387076, 1.000000000000000000, 0.8660254037844387076, 1.000000000000000000, 0.8660254037844387076, 1.000000000000000000, 0.8660254037844387076, 1.000000000000000000, 0.8660254037844387076, 1.000000000000000000, 0.8660254037844387076, 1.000000000000000000, 0.8660254037844387076, 1.000000000000000000, 0.8660254037844387076, 1.000000000000000000, 0.8660254037844387076, 1.000000000000000000, 0.8660254037844387076, 1.000000000000000000, 0.8660254037844387076, 1.000000000000000000, 0.8660254037844387076, 1.000000000000000000, 0.8660254037844387076, 1.000000000000000000, 0.8660254037844387076, 1.000000000000000000, 0.8660254037844387076, 1.000000000000000000, 0.8660254037844387076, 1.000000000000000000, 0.8660254037844387076, 1.000000000000000000, 0.8660254037844387076, 1.000000000000000000, 0.8660254037844387076, 1.000000000000000000, 0.8660254037844387076, 1.000000000000000000, 0.8660254037844387076, 1.000000000000000000, 0.8660254037844387076, 1.000000000000000000, 0.8660254037844387076, 1.000000000000000000, 0.8660254037844387076, 1.000000000000000000, 0.9111412529300411123, 0.9401537613649495473, 0.9401537613649495473, 0.9401537613649495473),
 ( 1.000000000000000000, 0.8660254037844387076, 1.000000000000000000, 0.8660254037844387076, 1.000000000000000000, 0.8660254037844387076, 1.000000000000000000, 0.8660254037844387076, 1.000000000000000000, 0.8660254037844387076, 1.000000000000000000, 0.8660254037844387076, 1.000000000000000000, 0.8660254037844387076, 1.000000000000000000, 0.8660254037844387076, 1.000000000000000000, 0.8660254037844387076, 1.000000000000000000, 0.8660254037844387076, 1.000000000000000000, 0.8660254037844387076, 1.000000000000000000, 0.8660254037844387076, 1.000000000000000000, 0.8660254037844387076, 1.000000000000000000, 0.8660254037844387076, 1.000000000000000000, 0.8660254037844387076, 1.000000000000000000, 0.8660254037844387076, 1.000000000000000000, 0.8660254037844387076, 1.000000000000000000, 0.8660254037844387076, 1.000000000000000000, 0.8660254037844387076, 1.000000000000000000, 0.8660254037844387076, 1.000000000000000000, 0.8660254037844387076, 1.000000000000000000, 0.8660254037844387076, 1.000000000000000000, 0.8660254037844387076, 1.000000000000000000, 0.8660254037844387076, 1.000000000000000000, 0.8660254037844387076, 1.000000000000000000, 0.8660254037844387076, 1.000000000000000000, 0.8660254037844387076, 1.000000000000000000, 0.8660254037844387076, 1.000000000000000000, 0.8660254037844387076, 1.000000000000000000, 0.8660254037844387076, 1.000000000000000000, 0.8660254037844387076, 1.000000000000000000, 0.8660254037844387076, 1.000000000000000000, 0.8660254037844387076, 1.000000000000000000, 0.8660254037844387076, 1.000000000000000000, 0.8660254037844387076, 1.000000000000000000, 0.8660254037844387076, 1.000000000000000000, 0.8660254037844387076, 1.000000000000000000, 0.8660254037844387076, 1.000000000000000000, 0.8660254037844387076, 1.000000000000000000, 0.8660254037844387076, 1.000000000000000000, 0.8660254037844387076, 1.000000000000000000, 0.8660254037844387076, 1.000000000000000000, 0.8660254037844387076, 1.000000000000000000, 0.8660254037844387076, 1.000000000000000000, 0.8660254037844387076, 1.000000000000000000, 0.8660254037844387076, 1.000000000000000000, 0.8660254037844387076, 1.000000000000000000, 0.8660254037844387076, 1.000000000000000000, 0.8660254037844387076, 1.000000000000000000, 0.8660254037844387076, 1.000000000000000000, 0.8660254037844387076, 1.000000000000000000, 0.8660254037844387076, 1.000000000000000000, 0.8660254037844387076, 1.000000000000000000, 0.8660254037844387076, 1.000000000000000000, 0.8660254037844387076, 1.000000000000000000, 0.8660254037844387076, 1.000000000000000000, 0.8660254037844387076, 1.000000000000000000, 0.8660254037844387076, 1.000000000000000000, 0.8660254037844387076, 1.000000000000000000, 0.8660254037844387076, 1.000000000000000000, 0.8660254037844387076, 1.000000000000000000, 0.8660254037844387076, 1.000000000000000000, 0.8660254037844387076, 1.000000000000000000, 0.8660254037844387076, 1.000000000000000000, 0.8660254037844387076, 1.000000000000000000, 0.8660254037844387076, 1.000000000000000000, 0.9111412529300411123, 0.9401537613649495473, 0.9401537613649495473, 0.9401537613649495473) ) ) 
 REPRESENTATION_ITEM ( '' )  SURFACE ( )  );
#6268=CARTESIAN_POINT ( 'NONE',  ( 1.128215178124999607, -0.7406249993854829849, -1.954126010382871259 ) ) ;
#6274=EDGE_CURVE ( 'NONE', #3142, #2494, #3791, .T. ) ;
#6275=CARTESIAN_POINT ( 'NONE',  ( 4.996790860652426159E-15, -1.856249998770965748, -2.500000000000000000 ) ) ;
#6280=CARTESIAN_POINT ( 'NONE',  ( 2.500000000000000000, -3.787499999999999645, -1.443375672974064994 ) ) ;
#6282=CARTESIAN_POINT ( 'NONE',  ( -0.6698729810778069060, -0.4861538093386316151, -2.500000000000000000 ) ) ;
#6283=CARTESIAN_POINT ( 'NONE',  ( -2.256430356250000102, -0.1406249993854829794, 0.000000000000000000 ) ) ;
#6289=EDGE_CURVE ( 'NONE', #3656, #7920, #3863, .T. ) ;
#6291=CARTESIAN_POINT ( 'NONE',  ( 2.256430356250000546, -4.903124999385481964, 1.302750673588579877 ) ) ;
#6294=CARTESIAN_POINT ( 'NONE',  ( 1.128215178124999607, -2.540624999385482585, -1.954126010382871259 ) ) ;
#6301=ORIENTED_EDGE ( 'NONE', *, *, #5449, .F. ) ;
#6303=VECTOR ( 'NONE', #4988, 1000.000000000000000 ) ;
#6306=ORIENTED_EDGE ( 'NONE', *, *, #5829, .F. ) ;
#6307=CARTESIAN_POINT ( 'NONE',  ( -1.128215178125000273, -3.478124999385482141, -1.954126010382871259 ) ) ;
#6308=ORIENTED_EDGE ( 'NONE', *, *, #7485, .F. ) ;
#6314=CARTESIAN_POINT ( 'NONE',  ( 1.128215178124999607, -0.8531249993854828073, -1.954126010382871259 ) ) ;
#6319=CARTESIAN_POINT ( 'NONE',  ( -2.500000000000000000, -2.681249998770965259, -1.443375672974064106 ) ) ;
#6320=CARTESIAN_POINT ( 'NONE',  ( 1.045839947578414805E-15, -0.9562499987709659477, -2.500000000000000000 ) ) ;
#6323=CARTESIAN_POINT ( 'NONE',  ( 1.128215178125001161, -1.340624999385482852, 1.954126010382870815 ) ) ;
#6326=VECTOR ( 'NONE', #10272, 1000.000000000000227 ) ;
#6332=CARTESIAN_POINT ( 'NONE',  ( 2.500000000000000000, -4.687500000000000000, -1.443375672974064994 ) ) ;
#6336=CARTESIAN_POINT ( 'NONE',  ( -2.256430356250000102, -3.403124999385482408, 0.000000000000000000 ) ) ;
#6343=CARTESIAN_POINT ( 'NONE',  ( -1.595409442497313560E-16, -3.403124999385482408, -2.605501347177161087 ) ) ;
#6346=CARTESIAN_POINT ( 'NONE',  ( -1.128215178124998497, -2.765624999385482674, 1.954126010382872147 ) ) ;
#6349=DIRECTION ( 'NONE',  ( 0.000000000000000000, -1.000000000000000000, 0.000000000000000000 ) ) ;
#6352=CARTESIAN_POINT ( 'NONE',  ( 2.500000000000000444, -3.356249998770965082, 1.443375672974063439 ) ) ;
#6356=CARTESIAN_POINT ( 'NONE',  ( -2.256430356250000102, -4.753124999385482496, 0.000000000000000000 ) ) ;
#6361=CARTESIAN_POINT ( 'NONE',  ( 2.500000000000000000, -1.087499999999999911, -1.443375672974065438 ) ) ;
#6362=CARTESIAN_POINT ( 'NONE',  ( 2.256430356250000546, -2.765624999385482674, 1.302750673588579877 ) ) ;
#6366=CARTESIAN_POINT ( 'NONE',  ( -2.500000000000000000, -2.193749998770965881, 0.000000000000000000 ) ) ;
#6367=VECTOR ( 'NONE', #5208, 1000.000000000000000 ) ;
#6369=CARTESIAN_POINT ( 'NONE',  ( -0.6698729810778054627, -3.057596189432333578, 2.500000000000000000 ) ) ;
#6370=DIRECTION ( 'NONE',  ( 0.000000000000000000, 0.000000000000000000, -1.000000000000000000 ) ) ;
#6371=CARTESIAN_POINT ( 'NONE',  ( 2.256430356250000102, -4.865624999385482319, -2.763330213280484622E-16 ) ) ;
#6378=CARTESIAN_POINT ( 'NONE',  ( 1.250000000000001110, -4.349999999999999645, 2.165063509461096380 ) ) ;
#6381=CARTESIAN_POINT ( 'NONE',  ( -1.128215178124998497, -3.778124999385482408, 1.954126010382872147 ) ) ;
#6388=VECTOR ( 'NONE', #8314, 1000.000000000000000 ) ;
#6390=CARTESIAN_POINT ( 'NONE',  ( 1.128215178125001161, -4.490624999385482319, 1.954126010382870815 ) ) ;
#6392=EDGE_LOOP ( 'NONE', ( #1706, #3924, #6583, #9466 ) ) ;
#6394=CARTESIAN_POINT ( 'NONE',  ( -1.128215178124998497, -1.865624999385482763, 1.954126010382872147 ) ) ;
#6401=DIRECTION ( 'NONE',  ( 0.000000000000000000, -1.000000000000000000, 0.000000000000000000 ) ) ;
#6404=CARTESIAN_POINT ( 'NONE',  ( -2.256430356250000102, -3.440624999385482496, -1.302750673588580321 ) ) ;
#6405=CARTESIAN_POINT ( 'NONE',  ( 1.034219503716432668E-14, -5.006249998770964993, -2.500000000000000000 ) ) ;
#6406=AXIS2_PLACEMENT_3D ( 'NONE', #6580, #7267, #9771 ) ;
#6411=CARTESIAN_POINT ( 'NONE',  ( -2.256430356250000102, -4.753124999385482496, 0.000000000000000000 ) ) ;
#6417=CARTESIAN_POINT ( 'NONE',  ( 1.250000000000001110, -3.393749998770965615, 2.165063509461096380 ) ) ;
#6418=EDGE_CURVE ( 'NONE', #2954, #3286, #4856, .T. ) ;
#6422=CARTESIAN_POINT ( 'NONE',  ( -2.256430356250000102, -5.090624999385482852, 0.000000000000000000 ) ) ;
#6423=EDGE_LOOP ( 'NONE', ( #2221, #3505, #10214, #4000 ) ) ;
#6433=CARTESIAN_POINT ( 'NONE',  ( 4.786228327491941173E-16, -3.740624999385482319, 2.605501347177161087 ) ) ;
#6441=LINE ( 'NONE', #10323, #1462 ) ;
#6442=CARTESIAN_POINT ( 'NONE',  ( 1.128215178124999607, -3.890624999385482674, -1.954126010382871259 ) ) ;
#6444=ORIENTED_EDGE ( 'NONE', *, *, #8074, .F. ) ;
#6447=CARTESIAN_POINT ( 'NONE',  ( 2.256430356250000102, -2.165624999385483029, -2.763330213280484622E-16 ) ) ;
#6453=EDGE_CURVE ( 'NONE', #7399, #5471, #5112, .T. ) ;
#6454=CARTESIAN_POINT ( 'NONE',  ( 2.500000000000000444, -3.412500000000000089, 1.443375672974063439 ) ) ;
#6462=CARTESIAN_POINT ( 'NONE',  ( 0.2187216588148096774, -20.00000000000000000, 3.085264589354759224 ) ) ;
#6463=CARTESIAN_POINT ( 'NONE',  ( -2.256430356250000102, -2.990624999385482763, -1.302750673588580321 ) ) ;
#6467=CARTESIAN_POINT ( 'NONE',  ( 2.500000000000000000, -4.668749998770964638, -3.061616997868383141E-16 ) ) ;
#6468=ORIENTED_EDGE ( 'NONE', *, *, #6527, .F. ) ;
#6470=CARTESIAN_POINT ( 'NONE',  ( 2.500000000000000000, -1.031249998770965792, -1.443375672974065438 ) ) ;
#6473=CARTESIAN_POINT ( 'NONE',  ( 4.786228327491941173E-16, -4.528124999385482852, 2.605501347177161087 ) ) ;
#6477=DIRECTION ( 'NONE',  ( 0.000000000000000000, -1.000000000000000000, 0.000000000000000000 ) ) ;
#6479=CARTESIAN_POINT ( 'NONE',  ( 2.500000000000000000, -1.968749998770965792, -3.061616997868383141E-16 ) ) ;
#6484=CARTESIAN_POINT ( 'NONE',  ( -1.595409442497313560E-16, -3.515624999385482674, -2.605501347177161087 ) ) ;
#6489=CARTESIAN_POINT ( 'NONE',  ( -9.703070624755296135E-15, -4.837500000000001243, 2.500000000000000444 ) ) ;
#6491=CARTESIAN_POINT ( 'NONE',  ( 2.256430356250000546, -4.453124999385482674, 1.302750673588579877 ) ) ;
#6495=CARTESIAN_POINT ( 'NONE',  ( 4.786228327491941173E-16, -4.078124999385482674, 2.605501347177161087 ) ) ;
#6502=CARTESIAN_POINT ( 'NONE',  ( 0.6698729810778025762, -3.467403810567665445, 2.500000000000002665 ) ) ;
#6505=CARTESIAN_POINT ( 'NONE',  ( 2.500000000000000444, -4.256249998770964993, 1.443375672974063439 ) ) ;
#6508=CARTESIAN_POINT ( 'NONE',  ( 1.128215178124999607, -3.553124999385482319, -1.954126010382871259 ) ) ;
#6513=CARTESIAN_POINT ( 'NONE',  ( 2.500000000000000000, -4.218749998770966236, -3.061616997868383141E-16 ) ) ;
#6515=CARTESIAN_POINT ( 'NONE',  ( -9.703070624755296135E-15, -5.231249998770965526, 2.500000000000000444 ) ) ;
#6519=CARTESIAN_POINT ( 'NONE',  ( -2.256430356250000102, -4.640624999385482674, 0.000000000000000000 ) ) ;
#6522=LINE ( 'NONE', #5697, #5324 ) ;
#6527=EDGE_CURVE ( 'NONE', #3372, #3656, #5740, .T. ) ;
#6528=DIRECTION ( 'NONE',  ( 0.000000000000000000, -1.000000000000000000, 0.000000000000000000 ) ) ;
#6534=ORIENTED_EDGE ( 'NONE', *, *, #181, .T. ) ;
#6535=CARTESIAN_POINT ( 'NONE',  ( 1.250000000000001110, -4.743749998770965703, 2.165063509461096380 ) ) ;
#6538=CARTESIAN_POINT ( 'NONE',  ( 3.486133158594717003E-16, -0.1125000000000000167, -2.500000000000000000 ) ) ;
#6541=CARTESIAN_POINT ( 'NONE',  ( -2.256430356250000102, -4.640624999385482674, 0.000000000000000000 ) ) ;
#6542=CARTESIAN_POINT ( 'NONE',  ( 3.061616997868383141E-16, 0.000000000000000000, 2.500000000000000000 ) ) ;
#6554=CARTESIAN_POINT ( 'NONE',  ( -2.256430356249998770, -4.265624999385482674, 1.302750673588581876 ) ) ;
#6560=CARTESIAN_POINT ( 'NONE',  ( -2.499999999999999556, -5.306249998770963927, 1.443375672974065882 ) ) ;
#6565=CARTESIAN_POINT ( 'NONE',  ( -2.256430356250000102, -3.778124999385482408, -1.302750673588580321 ) ) ;
#6568=ADVANCED_FACE ( 'NONE', ( #7132 ), #8714, .T. ) ;
#6569=EDGE_CURVE ( 'NONE', #2184, #3756, #7921, .T. ) ;
#6570=CARTESIAN_POINT ( 'NONE',  ( 0.6698729810778087934, -1.482596189432334288, -2.499999999999999112 ) ) ;
#6572=CARTESIAN_POINT ( 'NONE',  ( 2.500000000000000000, -3.731249998770965970, -1.443375672974065438 ) ) ;
#6580=CARTESIAN_POINT ( 'NONE',  ( 0.000000000000000000, 0.000000000000000000, 0.000000000000000000 ) ) ;
#6582=CARTESIAN_POINT ( 'NONE',  ( 2.500000000000000000, -4.724999999999998757, -3.061616997868383141E-16 ) ) ;
#6583=ORIENTED_EDGE ( 'NONE', *, *, #5758, .T. ) ;
#6585=CARTESIAN_POINT ( 'NONE',  ( -2.256430356249999214, -5.053124999385482319, 1.302750673588581876 ) ) ;
#6590=CARTESIAN_POINT ( 'NONE',  ( -2.499999999999999112, -0.8624999999999998224, 1.443375672974065882 ) ) ;
#6596=ORIENTED_EDGE ( 'NONE', *, *, #512, .T. ) ;
#6603=VECTOR ( 'NONE', #9056, 1000.000000000000000 ) ;
#6604=CARTESIAN_POINT ( 'NONE',  ( -1.728529299398585906, -5.253648441416169490, -1.450401466387756244 ) ) ;
#6606=CARTESIAN_POINT ( 'NONE',  ( 5.302876193624534821E-16, -4.331249998770966059, 2.886751345948128655 ) ) ;
#6608=ORIENTED_EDGE ( 'NONE', *, *, #9528, .T. ) ;
#6615=CARTESIAN_POINT ( 'NONE',  ( -2.500000000000000000, -3.600000000000000089, 0.000000000000000000 ) ) ;
#6618=AXIS2_PLACEMENT_3D ( 'NONE', #9376, #687, #4668 ) ;
#6619=CARTESIAN_POINT ( 'NONE',  ( 0.000000000000000000, -20.00000000000000000, 0.000000000000000000 ) ) ;
#6634=CARTESIAN_POINT ( 'NONE',  ( 2.500000000000000000, -0.2250000000000000056, -3.061616997868383141E-16 ) ) ;
#6635=CARTESIAN_POINT ( 'NONE',  ( 1.034219503716432668E-14, -2.812500000000000444, -2.500000000000000000 ) ) ;
#6637=B_SPLINE_CURVE_WITH_KNOTS ( 'NONE', 1,
 ( #8430, #7756 ),
 .UNSPECIFIED., .F., .F.,
 ( 2, 2 ),
 ( 0.000000000000000000, 1.000000000000000000 ),
 .UNSPECIFIED. ) ;
#6640=CARTESIAN_POINT ( 'NONE',  ( -1.728529299398585906, -5.253648441416169490, -1.450401466387756244 ) ) ;
#6645=( BOUNDED_CURVE ( )  B_SPLINE_CURVE ( 2, ( #6320, #3281, #27, #6470, #7938, #1552, #3231, #4792, #8676 ),
 .UNSPECIFIED., .F., .T. ) 
 B_SPLINE_CURVE_WITH_KNOTS ( ( 3, 2, 2, 2, 3 ),
 ( 0.1041666666666666713, 0.1111111111111111049, 0.1250000000000000000, 0.1388888888888888951, 0.1458333333333333426 ),
 .UNSPECIFIED. ) 
 CURVE ( )  GEOMETRIC_REPRESENTATION_ITEM ( )  RATIONAL_B_SPLINE_CURVE ( ( 0.9330127018922194093, 0.9330127018922194093, 1.000000000000000000, 0.8660254037844387076, 1.000000000000000000, 0.8660254037844387076, 1.000000000000000000, 0.9330127018922194093, 0.9330127018922194093 ) ) 
 REPRESENTATION_ITEM ( '' )  );
#6647=EDGE_CURVE ( 'NONE', #4141, #4703, #9069, .T. ) ;
#6657=CARTESIAN_POINT ( 'NONE',  ( -2.500000000000000000, -4.443749998770965881, 0.000000000000000000 ) ) ;
#6661=CARTESIAN_POINT ( 'NONE',  ( -1.085030467718112069E-15, -15.00000000000000000, 3.464101615137756163 ) ) ;
#6675=CYLINDRICAL_SURFACE ( 'NONE', #8446, 2.500000000000000000 ) ;
#6679=DIRECTION ( 'NONE',  ( 0.000000000000000000, -1.000000000000000000, 0.000000000000000000 ) ) ;
#6683=CARTESIAN_POINT ( 'NONE',  ( -2.499999999999999556, -0.4124999999999999778, 1.443375672974065882 ) ) ;
#6690=DIRECTION ( 'NONE',  ( 0.000000000000000000, 0.000000000000000000, -1.000000000000000000 ) ) ;
#6705=CARTESIAN_POINT ( 'NONE',  ( -2.256430356250000102, -2.053124999385482763, 0.000000000000000000 ) ) ;
#6723=CARTESIAN_POINT ( 'NONE',  ( -9.703070624755296135E-15, -4.837500000000001243, 2.500000000000000444 ) ) ;
#6732=CARTESIAN_POINT ( 'NONE',  ( -2.499999999999999112, -0.4124999999999999223, 1.443375672974065882 ) ) ;
#6733=CARTESIAN_POINT ( 'NONE',  ( 0.000000000000000000, 0.000000000000000000, 0.000000000000000000 ) ) ;
#6734=CARTESIAN_POINT ( 'NONE',  ( 0.000000000000000000, 0.000000000000000000, -2.500000000000000000 ) ) ;
#6735=CARTESIAN_POINT ( 'NONE',  ( -2.500000000000000000, -2.287499999999999645, -1.443375672974064106 ) ) ;
#6737=CARTESIAN_POINT ( 'NONE',  ( -1.249999999999998224, -1.724999999999999645, 2.165063509461097713 ) ) ;
#6743=CARTESIAN_POINT ( 'NONE',  ( -1.250000000000000222, -0.9749999999999999778, -2.165063509461096825 ) ) ;
#6744=ORIENTED_EDGE ( 'NONE', *, *, #4960, .T. ) ;
#6750=CARTESIAN_POINT ( 'NONE',  ( -1.128215178124998497, -0.5156249993854828961, 1.954126010382872147 ) ) ;
#6753=CARTESIAN_POINT ( 'NONE',  ( 9.877377282685029372E-16, -0.7874999999999998668, 2.500000000000000000 ) ) ;
#6755=CARTESIAN_POINT ( 'NONE',  ( 0.000000000000000000, 0.000000000000000000, 0.000000000000000000 ) ) ;
#6759=CARTESIAN_POINT ( 'NONE',  ( 2.256430356250000102, -1.828124999385482674, -2.763330213280484622E-16 ) ) ;
#6760=ORIENTED_EDGE ( 'NONE', *, *, #512, .F. ) ;
#6769=FACE_OUTER_BOUND ( 'NONE', #3189, .T. ) ;
#6772=ORIENTED_EDGE ( 'NONE', *, *, #10299, .T. ) ;
#6778=ORIENTED_EDGE ( 'NONE', *, *, #3277, .F. ) ;
#6784=ORIENTED_EDGE ( 'NONE', *, *, #42, .T. ) ;
#6787=ORIENTED_EDGE ( 'NONE', *, *, #9948, .F. ) ;
#6788=VECTOR ( 'NONE', #609, 1000.000000000000114 ) ;
#6789=CARTESIAN_POINT ( 'NONE',  ( 2.500000000000000444, -0.7124999999999999112, 1.443375672974063439 ) ) ;
#6792=CARTESIAN_POINT ( 'NONE',  ( 1.128215178125001161, -1.903124999385482852, 1.954126010382870815 ) ) ;
#6794=CARTESIAN_POINT ( 'NONE',  ( 1.249999999999999334, -0.5437499987709658589, -2.165063509461096825 ) ) ;
#6798=( LENGTH_UNIT ( ) NAMED_UNIT ( * ) SI_UNIT ( .MILLI., .METRE. ) );
#6810=VERTEX_POINT ( 'NONE', #1151 ) ;
#6811=DIRECTION ( 'NONE',  ( 0.000000000000000000, 0.000000000000000000, -1.000000000000000000 ) ) ;
#6812=CARTESIAN_POINT ( 'NONE',  ( -1.128215178124998497, -2.428124999385482763, 1.954126010382872147 ) ) ;
#6815=VECTOR ( 'NONE', #2668, 1000.000000000000000 ) ;
#6827=CARTESIAN_POINT ( 'NONE',  ( -2.781278341185190239, -20.00000000000000000, -1.353213781785880476 ) ) ;
#6829=CARTESIAN_POINT ( 'NONE',  ( -1.249999999999998224, -0.7687499987709658367, 2.165063509461097713 ) ) ;
#6832=EDGE_CURVE ( 'NONE', #3838, #9728, #418, .T. ) ;
#6841=CARTESIAN_POINT ( 'NONE',  ( -1.249999999999998224, -0.8249999999999998446, 2.165063509461097713 ) ) ;
#6843=CARTESIAN_POINT ( 'NONE',  ( 0.000000000000000000, -20.00000000000000000, -2.500000000000000444 ) ) ;
#6844=CARTESIAN_POINT ( 'NONE',  ( -1.595409442497313560E-16, -1.265624999385482896, -2.605501347177161087 ) ) ;
#6853=CARTESIAN_POINT ( 'NONE',  ( 4.786228327491940187E-16, -1.828124999385482674, 2.605501347177161087 ) ) ;
#6854=PLANE ( 'NONE',  #2456 ) ;
#6859=ORIENTED_EDGE ( 'NONE', *, *, #9357, .T. ) ;
#6867=CARTESIAN_POINT ( 'NONE',  ( -1.595409442497313560E-16, -1.715624999385482630, -2.605501347177161087 ) ) ;
#6872=CARTESIAN_POINT ( 'NONE',  ( -1.128215178124998497, -1.978124999385482807, 1.954126010382872147 ) ) ;
#6878=LINE ( 'NONE', #1394, #6788 ) ;
#6882=CARTESIAN_POINT ( 'NONE',  ( 2.256430356249999658, -0.7781249993854829627, -1.302750673588581432 ) ) ;
#6894=CARTESIAN_POINT ( 'NONE',  ( 2.500000000000000000, -0.6374999999999999556, -1.443375672974064994 ) ) ;
#6896=CARTESIAN_POINT ( 'NONE',  ( 2.500000000000000000, -2.381249998770965437, -1.443375672974065438 ) ) ;
#6898=CARTESIAN_POINT ( 'NONE',  ( 1.128215178124999607, -2.653124999385482408, -1.954126010382871259 ) ) ;
#6904=CARTESIAN_POINT ( 'NONE',  ( 2.500000000000000000, -1.987499999999999600, -1.443375672974065438 ) ) ;
#6907=CARTESIAN_POINT ( 'NONE',  ( 0.000000000000000000, 0.000000000000000000, 0.000000000000000000 ) ) ;
#6908=ORIENTED_EDGE ( 'NONE', *, *, #7239, .T. ) ;
#6909=CARTESIAN_POINT ( 'NONE',  ( -1.595409442497313560E-16, -0.7031249993854830072, -2.605501347177161087 ) ) ;
#6912=CARTESIAN_POINT ( 'NONE',  ( -0.6698729810778054627, -1.201346188203299858, 2.500000000000000000 ) ) ;
#6914=CARTESIAN_POINT ( 'NONE',  ( 1.034219503716432668E-14, -3.262500000000000178, -2.500000000000000000 ) ) ;
#6920=DIRECTION ( 'NONE',  ( -0.000000000000000000, -1.000000000000000000, -0.000000000000000000 ) ) ;
#6921=CARTESIAN_POINT ( 'NONE',  ( -2.256430356250000102, -1.190624999385482941, -1.302750673588580321 ) ) ;
#6927=CARTESIAN_POINT ( 'NONE',  ( 2.256430356250000102, -1.828124999385482674, -2.763330213280484622E-16 ) ) ;
#6928=( BOUNDED_CURVE ( )  B_SPLINE_CURVE ( 2, ( #5266, #4484, #6048, #6104, #8408, #9926, #617, #457, #1239 ),
 .UNSPECIFIED., .F., .F. ) 
 B_SPLINE_CURVE_WITH_KNOTS ( ( 3, 2, 2, 2, 3 ),
 ( 0.6458333333333333703, 0.6527777777777777901, 0.6666666666666666297, 0.6805555555555555802, 0.6875000000000000000 ),
 .UNSPECIFIED. ) 
 CURVE ( )  GEOMETRIC_REPRESENTATION_ITEM ( )  RATIONAL_B_SPLINE_CURVE ( ( 0.9330127018922192983, 0.9330127018922198534, 1.000000000000000000, 0.8660254037844387076, 1.000000000000000000, 0.8660254037844387076, 1.000000000000000000, 0.9330127018922194093, 0.9330127018922194093 ) ) 
 REPRESENTATION_ITEM ( '' )  );
#6932=CARTESIAN_POINT ( 'NONE',  ( 1.249999999999999334, -0.9937499987709658145, -2.165063509461096825 ) ) ;
#6934=CARTESIAN_POINT ( 'NONE',  ( 0.000000000000000000, 0.000000000000000000, 0.000000000000000000 ) ) ;
#6936=LINE ( 'NONE', #6154, #9742 ) ;
#6937=CARTESIAN_POINT ( 'NONE',  ( 9.877377282685029372E-16, -4.387499999999999289, 2.500000000000000000 ) ) ;
#6938=CARTESIAN_POINT ( 'NONE',  ( -2.256430356250000102, -2.428124999385482319, -1.302750673588580321 ) ) ;
#6939=CARTESIAN_POINT ( 'NONE',  ( 3.061616997868383141E-16, 0.000000000000000000, 2.500000000000000000 ) ) ;
#6940=VECTOR ( 'NONE', #6477, 1000.000000000000000 ) ;
#6944=DIRECTION ( 'NONE',  ( -0.000000000000000000, 1.000000000000000000, -0.000000000000000000 ) ) ;
#6952=CARTESIAN_POINT ( 'NONE',  ( -2.499999999999999556, -4.912499999999998757, 1.443375672974065882 ) ) ;
#6955=CARTESIAN_POINT ( 'NONE',  ( -2.256430356250000102, -1.153124999385482852, 0.000000000000000000 ) ) ;
#6961=CARTESIAN_POINT ( 'NONE',  ( -0.6698729810778020211, -3.186153809338631238, -2.500000000000002665 ) ) ;
#6965=ORIENTED_EDGE ( 'NONE', *, *, #7604, .F. ) ;
#6966=CARTESIAN_POINT ( 'NONE',  ( 2.256430356250000102, -0.8156249993854829405, -2.763330213280484622E-16 ) ) ;
#6969=FACE_OUTER_BOUND ( 'NONE', #7071, .T. ) ;
#6979=EDGE_CURVE ( 'NONE', #8050, #6810, #1962, .T. ) ;
#6980=CARTESIAN_POINT ( 'NONE',  ( -1.128215178124998497, -3.328124999385482230, 1.954126010382872147 ) ) ;
#6981=EDGE_LOOP ( 'NONE', ( #8333, #9810, #2671, #7708 ) ) ;
#6985=CARTESIAN_POINT ( 'NONE',  ( 1.128215178124999607, -1.753124999385482718, -1.954126010382871259 ) ) ;
#6992=( BOUNDED_CURVE ( )  B_SPLINE_CURVE ( 2, ( #5126, #2835, #1206, #1156, #5290, #4345, #478, #3563, #8486 ),
 .UNSPECIFIED., .F., .T. ) 
 B_SPLINE_CURVE_WITH_KNOTS ( ( 3, 2, 2, 2, 3 ),
 ( 0.7291666666666667407, 0.7361111111111111605, 0.7500000000000000000, 0.7638888888888888395, 0.7708333333333333703 ),
 .UNSPECIFIED. ) 
 CURVE ( )  GEOMETRIC_REPRESENTATION_ITEM ( )  RATIONAL_B_SPLINE_CURVE ( ( 0.9330127018922192983, 0.9330127018922198534, 1.000000000000000000, 0.8660254037844387076, 1.000000000000000000, 0.8660254037844387076, 1.000000000000000000, 0.9330127018922187432, 0.9330127018922192983 ) ) 
 REPRESENTATION_ITEM ( '' )  );
#6995=CARTESIAN_POINT ( 'NONE',  ( 2.256430356250000546, -1.753124999385482718, 1.302750673588579877 ) ) ;
#6997=CARTESIAN_POINT ( 'NONE',  ( -1.250000000000000222, -0.9187499987709658589, -2.165063509461096825 ) ) ;
#7003=ORIENTED_EDGE ( 'NONE', *, *, #8620, .T. ) ;
#7004=CARTESIAN_POINT ( 'NONE',  ( -2.500000000000000000, -4.949999999999999289, 0.000000000000000000 ) ) ;
#7005=AXIS2_PLACEMENT_3D ( 'NONE', #7306, #880, #238 ) ;
#7007=CARTESIAN_POINT ( 'NONE',  ( 2.256430356250000546, -1.415624999385482807, 1.302750673588579877 ) ) ;
#7016=CARTESIAN_POINT ( 'NONE',  ( 1.128215178124999607, -1.640624999385482896, -1.954126010382871259 ) ) ;
#7020=CARTESIAN_POINT ( 'NONE',  ( -1.595409442497313560E-16, -1.153124999385483074, -2.605501347177161087 ) ) ;
#7027=ORIENTED_EDGE ( 'NONE', *, *, #10290, .T. ) ;
#7031=CARTESIAN_POINT ( 'NONE',  ( 4.786228327491941173E-16, -5.090624999385482852, 2.605501347177161087 ) ) ;
#7032=ORIENTED_EDGE ( 'NONE', *, *, #1705, .T. ) ;
#7036=CARTESIAN_POINT ( 'NONE',  ( 2.500000000000000000, -0.2250000000000000056, -3.061616997868383141E-16 ) ) ;
#7038=CARTESIAN_POINT ( 'NONE',  ( -1.595409442497313560E-16, -2.615624999385482319, -2.605501347177161087 ) ) ;
#7042=CARTESIAN_POINT ( 'NONE',  ( -1.249999999999998224, -1.668749998770965970, 2.165063509461097713 ) ) ;
#7045=CARTESIAN_POINT ( 'NONE',  ( -9.703070624755296135E-15, -4.331249998770966059, 2.500000000000000444 ) ) ;
#7046=CARTESIAN_POINT ( 'NONE',  ( -2.256430356250000102, -1.078124999385482896, -1.302750673588580321 ) ) ;
#7047=ORIENTED_EDGE ( 'NONE', *, *, #9051, .T. ) ;
#7056=ORIENTED_EDGE ( 'NONE', *, *, #9765, .T. ) ;
#7057=CARTESIAN_POINT ( 'NONE',  ( 5.302876193624534821E-16, -3.937500000000000444, 2.886751345948128655 ) ) ;
#7059=CARTESIAN_POINT ( 'NONE',  ( -1.595409442497313560E-16, -3.965624999385482408, -2.605501347177161087 ) ) ;
#7062=PRODUCT_DEFINITION_CONTEXT ( 'detailed design', #865, 'design' ) ;
#7069=CARTESIAN_POINT ( 'NONE',  ( -1.128215178125000273, -2.465624999385482852, -1.954126010382871259 ) ) ;
#7071=EDGE_LOOP ( 'NONE', ( #4368, #8839, #1798, #515, #8129, #6222, #6772, #4512, #2164, #9461, #4433, #9566, #3845, #1269, #7047, #9230, #1587, #5725, #3085, #8569, #5444, #10180, #5958, #160, #8623, #3128 ) ) ;
#7072=CARTESIAN_POINT ( 'NONE',  ( -1.128215178125000273, -2.465624999385482852, -1.954126010382871259 ) ) ;
#7074=VECTOR ( 'NONE', #7874, 1000.000000000000000 ) ;
#7080=ORIENTED_EDGE ( 'NONE', *, *, #8510, .F. ) ;
#7084=CARTESIAN_POINT ( 'NONE',  ( -1.128215178124998497, -3.778124999385482408, 1.954126010382872147 ) ) ;
#7085=ORIENTED_EDGE ( 'NONE', *, *, #562, .F. ) ;
#7087=CARTESIAN_POINT ( 'NONE',  ( 9.877377282685029372E-16, -1.687499999999999778, 2.500000000000000000 ) ) ;
#7088=EDGE_CURVE ( 'NONE', #10177, #1260, #8699, .T. ) ;
#7089=CARTESIAN_POINT ( 'NONE',  ( -2.256430356250000102, -0.2906249993854829183, -1.302750673588580321 ) ) ;
#7091=ORIENTED_EDGE ( 'NONE', *, *, #8252, .T. ) ;
#7094=CARTESIAN_POINT ( 'NONE',  ( 2.500000000000000000, -1.068749998770965881, -3.061616997868383141E-16 ) ) ;
#7096=CARTESIAN_POINT ( 'NONE',  ( 6.123233995736709336E-17, 0.000000000000000000, 0.4999999999999953371 ) ) ;
#7098=CARTESIAN_POINT ( 'NONE',  ( -2.499999999999999112, -4.406249998770965348, 1.443375672974065882 ) ) ;
#7099=CARTESIAN_POINT ( 'NONE',  ( -1.595409442497313560E-16, -1.603124999385482807, -2.605501347177161087 ) ) ;
#7102=LINE ( 'NONE', #4022, #6940 ) ;
#7106=ORIENTED_EDGE ( 'NONE', *, *, #5617, .T. ) ;
#7112=CARTESIAN_POINT ( 'NONE',  ( -2.500000000000000000, -3.637499999999999734, -1.443375672974064106 ) ) ;
#7115=CARTESIAN_POINT ( 'NONE',  ( 1.128215178124999607, -3.553124999385482319, -1.954126010382871259 ) ) ;
#7122=CARTESIAN_POINT ( 'NONE',  ( -2.256430356250000102, -2.840624999385482852, 0.000000000000000000 ) ) ;
#7125=CARTESIAN_POINT ( 'NONE',  ( 4.786228327491941173E-16, -3.178124999385482763, 2.605501347177161087 ) ) ;
#7127=CYLINDRICAL_SURFACE ( 'NONE', #4588, 2.500000000000000000 ) ;
#7129=CARTESIAN_POINT ( 'NONE',  ( 2.500000000000000000, -3.281249998770965792, -1.443375672974065438 ) ) ;
#7132=FACE_OUTER_BOUND ( 'NONE', #9152, .T. ) ;
#7134=VERTEX_POINT ( 'NONE', #1572 ) ;
#7135=CARTESIAN_POINT ( 'NONE',  ( -1.128215178125000273, -3.928124999385483207, -1.954126010382871259 ) ) ;
#7141=CARTESIAN_POINT ( 'NONE',  ( 4.786228327491940187E-16, -4.190624999385482496, 2.605501347177161087 ) ) ;
#7147=CARTESIAN_POINT ( 'NONE',  ( 2.500000000000000000, -3.281249998770965792, -1.443375672974064994 ) ) ;
#7148=ORIENTED_EDGE ( 'NONE', *, *, #5503, .F. ) ;
#7152=CARTESIAN_POINT ( 'NONE',  ( 1.128215178124999607, -4.790624999385483029, -1.954126010382871259 ) ) ;
#7154=ORIENTED_EDGE ( 'NONE', *, *, #3072, .F. ) ;
#7161=AXIS2_PLACEMENT_3D ( 'NONE', #9932, #8360, #1915 ) ;
#7163=CARTESIAN_POINT ( 'NONE',  ( -2.500000000000000000, -4.087500000000000355, -1.443375672974064106 ) ) ;
#7164=CARTESIAN_POINT ( 'NONE',  ( -2.500000000000000000, -0.4312499987709658700, -1.443375672974064106 ) ) ;
#7165=CARTESIAN_POINT ( 'NONE',  ( 2.256430356250000102, -4.978124999385482141, -2.763330213280484622E-16 ) ) ;
#7175=CARTESIAN_POINT ( 'NONE',  ( 1.128215178124999607, -4.340624999385482852, -1.954126010382871259 ) ) ;
#7178=CARTESIAN_POINT ( 'NONE',  ( 4.786228327491941173E-16, -1.378124999385482941, 2.605501347177161087 ) ) ;
#7185=CARTESIAN_POINT ( 'NONE',  ( -2.500000000000000000, -0.1968749993854829461, 0.000000000000000000 ) ) ;
#7186=ORIENTED_EDGE ( 'NONE', *, *, #191, .F. ) ;
#7187=CARTESIAN_POINT ( 'NONE',  ( -2.256430356249999214, -3.365624999385482319, 1.302750673588581876 ) ) ;
#7193=CARTESIAN_POINT ( 'NONE',  ( 1.128215178125001161, -3.253124999385482496, 1.954126010382870815 ) ) ;
#7197=CARTESIAN_POINT ( 'NONE',  ( 2.500000000000000444, -3.356249998770965082, 1.443375672974063439 ) ) ;
#7202=CARTESIAN_POINT ( 'NONE',  ( 1.128215178125001161, -4.940624999385482496, 1.954126010382870815 ) ) ;
#7205=CARTESIAN_POINT ( 'NONE',  ( -2.500000000000000000, -3.581249998770966059, -1.443375672974064106 ) ) ;
#7208=ORIENTED_EDGE ( 'NONE', *, *, #3581, .T. ) ;
#7212=CARTESIAN_POINT ( 'NONE',  ( 1.128215178125001161, -4.153124999385482852, 1.954126010382870815 ) ) ;
#7220=LINE ( 'NONE', #54, #621 ) ;
#7221=CARTESIAN_POINT ( 'NONE',  ( -1.128215178124998497, -4.565624999385482496, 1.954126010382872147 ) ) ;
#7225=CARTESIAN_POINT ( 'NONE',  ( -2.256430356250000102, -1.040624999385483029, 0.000000000000000000 ) ) ;
#7227=( NAMED_UNIT ( * ) SI_UNIT ( $, .STERADIAN. ) SOLID_ANGLE_UNIT ( ) );
#7228=DIRECTION ( 'NONE',  ( 0.000000000000000000, -1.000000000000000000, 0.000000000000000000 ) ) ;
#7230=CARTESIAN_POINT ( 'NONE',  ( 1.249999999999999334, -3.243749998770965259, -2.165063509461096825 ) ) ;
#7231=CARTESIAN_POINT ( 'NONE',  ( 1.034219503716432668E-14, -3.262500000000000178, -2.500000000000000000 ) ) ;
#7234=CARTESIAN_POINT ( 'NONE',  ( 2.500000000000000000, -5.118749998770964815, -3.061616997868383141E-16 ) ) ;
#7239=EDGE_CURVE ( 'NONE', #3171, #471, #9855, .T. ) ;
#7241=CARTESIAN_POINT ( 'NONE',  ( -1.595409442497313560E-16, -3.965624999385482408, -2.605501347177161087 ) ) ;
#7245=VECTOR ( 'NONE', #7980, 1000.000000000000000 ) ;
#7246=CARTESIAN_POINT ( 'NONE',  ( 1.249999999999999334, -4.143749998770966059, -2.165063509461096825 ) ) ;
#7251=CARTESIAN_POINT ( 'NONE',  ( 1.128215178125001161, -3.140624999385482674, 1.954126010382870815 ) ) ;
#7261=CARTESIAN_POINT ( 'NONE',  ( -1.728525935690056192, -5.253648612710515309, -1.450405475118361043 ) ) ;
#7267=DIRECTION ( 'NONE',  ( 0.000000000000000000, -1.000000000000000000, 0.000000000000000000 ) ) ;
#7268=ADVANCED_FACE ( 'NONE', ( #4180 ), #1240, .T. ) ;
#7270=DIRECTION ( 'NONE',  ( 0.000000000000000000, -1.000000000000000000, 0.000000000000000000 ) ) ;
#7271=CARTESIAN_POINT ( 'NONE',  ( 2.256430356250000546, -4.003124999385482496, 1.302750673588579877 ) ) ;
#7276=CARTESIAN_POINT ( 'NONE',  ( 2.256430356249999658, -3.928124999385482319, -1.302750673588581432 ) ) ;
#7287=CARTESIAN_POINT ( 'NONE',  ( -9.703070624755296135E-15, -5.231249998770965526, 2.500000000000000444 ) ) ;
#7288=CARTESIAN_POINT ( 'NONE',  ( 0.000000000000000000, 0.000000000000000000, -2.500000000000000000 ) ) ;
#7291=CARTESIAN_POINT ( 'NONE',  ( 2.256430356250000546, -3.665624999385482585, 1.302750673588579877 ) ) ;
#7296=ADVANCED_FACE ( 'NONE', ( #4379 ), #4431, .T. ) ;
#7298=CARTESIAN_POINT ( 'NONE',  ( -2.500000000000000000, -4.893749998770965171, 0.000000000000000000 ) ) ;
#7300=VECTOR ( 'NONE', #5737, 1000.000000000000114 ) ;
#7302=CARTESIAN_POINT ( 'NONE',  ( 3.000000000000000000, -15.00000000000000000, 1.732050807568879192 ) ) ;
#7304=CARTESIAN_POINT ( 'NONE',  ( 1.128215178124999607, -2.990624999385482763, -1.954126010382871259 ) ) ;
#7306=CARTESIAN_POINT ( 'NONE',  ( 0.000000000000000000, -25.00000000000000000, 0.000000000000000000 ) ) ;
#7312=( GEOMETRIC_REPRESENTATION_CONTEXT ( 3 ) GLOBAL_UNCERTAINTY_ASSIGNED_CONTEXT ( ( #791 ) ) GLOBAL_UNIT_ASSIGNED_CONTEXT ( ( #10331, #8804, #7227 ) ) REPRESENTATION_CONTEXT ( 'NONE', 'WORKASPACE' ) );
#7318=CARTESIAN_POINT ( 'NONE',  ( 0.6698729810778112359, -4.576346188203299192, -2.499999999999996447 ) ) ;
#7322=CARTESIAN_POINT ( 'NONE',  ( -0.6698729810778066840, -0.09240381056766579226, -2.500000000000000000 ) ) ;
#7323=CARTESIAN_POINT ( 'NONE',  ( 2.256430356250000102, -3.515624999385482674, -2.763330213280484622E-16 ) ) ;
#7324=( BOUNDED_CURVE ( )  B_SPLINE_CURVE ( 2, ( #10344, #1693, #20, #6361, #1541, #5379, #8570, #9351, #77 ),
 .UNSPECIFIED., .F., .F. ) 
 B_SPLINE_CURVE_WITH_KNOTS ( ( 3, 2, 2, 2, 3 ),
 ( 0.1875000000000000000, 0.1944444444444444475, 0.2083333333333333426, 0.2222222222222222099, 0.2291666666666666574 ),
 .UNSPECIFIED. ) 
 CURVE ( )  GEOMETRIC_REPRESENTATION_ITEM ( )  RATIONAL_B_SPLINE_CURVE ( ( 0.9330127018922194093, 0.9330127018922194093, 1.000000000000000000, 0.8660254037844387076, 1.000000000000000000, 0.8660254037844387076, 1.000000000000000000, 0.9330127018922194093, 0.9330127018922194093 ) ) 
 REPRESENTATION_ITEM ( '' )  );
#7330=CARTESIAN_POINT ( 'NONE',  ( 1.250000000000001110, -3.393749998770965615, 2.165063509461096380 ) ) ;
#7332=CARTESIAN_POINT ( 'NONE',  ( 3.061616997868383141E-16, 0.000000000000000000, 2.500000000000000000 ) ) ;
#7337=CARTESIAN_POINT ( 'NONE',  ( 4.786228327491940187E-16, -4.640624999385481786, 2.605501347177161087 ) ) ;
#7338=CARTESIAN_POINT ( 'NONE',  ( 2.500000000000000000, -2.418749998770965526, -3.061616997868383141E-16 ) ) ;
#7344=CARTESIAN_POINT ( 'NONE',  ( -2.499999999999999556, -3.956249998770965615, 1.443375672974065882 ) ) ;
#7346=DIRECTION ( 'NONE',  ( 0.000000000000000000, 0.000000000000000000, -1.000000000000000000 ) ) ;
#7349=CARTESIAN_POINT ( 'NONE',  ( 1.128215178125001161, -3.590624999385482408, 1.954126010382870815 ) ) ;
#7360=DIRECTION ( 'NONE',  ( 0.04357787137382919396, -0.9961946980917455452, 0.07547908730517351172 ) ) ;
#7362=DIRECTION ( 'NONE',  ( 0.000000000000000000, -1.000000000000000000, 0.000000000000000000 ) ) ;
#7365=ORIENTED_EDGE ( 'NONE', *, *, #5652, .T. ) ;
#7367=CARTESIAN_POINT ( 'NONE',  ( 1.128215178125001161, -3.590624999385482408, 1.954126010382870815 ) ) ;
#7369=CARTESIAN_POINT ( 'NONE',  ( -2.500000000000000000, -2.737499999999999822, -1.443375672974064106 ) ) ;
#7370=LINE ( 'NONE', #9878, #6388 ) ;
#7373=AXIS2_PLACEMENT_3D ( 'NONE', #2241, #5998, #4533 ) ;
#7377=ORIENTED_EDGE ( 'NONE', *, *, #3276, .T. ) ;
#7384=CARTESIAN_POINT ( 'NONE',  ( 4.996790860652426159E-15, -2.306249998770965259, -2.500000000000000000 ) ) ;
#7387=AXIS2_PLACEMENT_3D ( 'NONE', #1103, #270, #7531 ) ;
#7388=CARTESIAN_POINT ( 'NONE',  ( 2.500000000000000000, -4.181249998770965703, -1.443375672974064994 ) ) ;
#7390=EDGE_CURVE ( 'NONE', #8910, #3336, #1651, .T. ) ;
#7399=VERTEX_POINT ( 'NONE', #9471 ) ;
#7404=DIRECTION ( 'NONE',  ( 0.000000000000000000, -1.000000000000000000, 0.000000000000000000 ) ) ;
#7416=CARTESIAN_POINT ( 'NONE',  ( -1.595409442497313560E-16, -4.753124999385481608, -2.605501347177161087 ) ) ;
#7417=PRESENTATION_STYLE_ASSIGNMENT (( #257 ) ) ;
#7419=CARTESIAN_POINT ( 'NONE',  ( 1.128215178124999607, -0.4031249993854829627, -1.954126010382871259 ) ) ;
#7428=CYLINDRICAL_SURFACE ( 'NONE', #7387, 2.500000000000000000 ) ;
#7430=CARTESIAN_POINT ( 'NONE',  ( -1.128215178124998497, -5.128124999385482496, 1.954126010382872147 ) ) ;
#7434=( BOUNDED_CURVE ( )  B_SPLINE_CURVE ( 2, ( #9206, #10221, #635, #2206, #689, #3779, #8652, #586, #477, #2263, #5289, #6070, #1364, #5408, #9261, #6909, #8601, #2152, #6966, #1474, #2094, #1314, #3052, #6017, #4558, #534, #6180, #6234, #7755, #9378, #10167, #3004, #1424, #3673, #7697, #5229, #4612, #5462, #9435, #9320, #7016, #5351, #7806, #2034, #4450, #6853, #8429, #3727, #3834, #10107, #1261, #2943, #4669, #6125, #10049, #8485, #7860, #7637, #2886, #4504, #8541, #3881, #7069, #2834, #5559, #1726, #4821, #2468, #8703, #3, #1628, #3937, #7122, #10325, #8017, #3302, #5513, #9633, #9583, #5663, #3160, #1680, #1524, #8852, #4873, #2414, #8063, #6343, #848, #4766, #2313, #897, #4140, #8115, #55, #5713, #4717, #7963, #7910, #799, #6442, #4086, #8751, #7271, #1575, #743, #110, #946, #9538, #2362, #3990, #3206, #7175, #4918, #4038, #6491, #6390, #5610, #7221, #8799, #3254, #9490, #9682, #2522, #8900, #10275, #3109, #6291, #5008, #9098, #8946, #2713, #1916, #9826, #5902 ),
 .UNSPECIFIED., .F., .F. ) 
 B_SPLINE_CURVE_WITH_KNOTS ( ( 3, 2, 2, 2, 2, 2, 2, 2, 2, 2, 2, 2, 2, 2, 2, 2, 2, 2, 2, 2, 2, 2, 2, 2, 2, 2, 2, 2, 2, 2, 2, 2, 2, 2, 2, 2, 2, 2, 2, 2, 2, 2, 2, 2, 2, 2, 2, 2, 2, 2, 2, 2, 2, 2, 2, 2, 2, 2, 2, 2, 2, 2, 2, 2, 2, 2, 2, 3 ),
 ( 0.000000000000000000, 0.01500076742380700850, 0.03000153484761401701, 0.04500230227142102551, 0.06000306969522803402, 0.07500383711903504946, 0.09000460454284205103, 0.1050053719666490665, 0.1200061393904560680, 0.1350069068142630835, 0.1500076742380700989, 0.1650084416618771144, 0.1800092090856841021, 0.1950099765094911175, 0.2100107439332981329, 0.2250115113571051484, 0.2400122787809121361, 0.2550130462047191515, 0.2700138136285261670, 0.2850145810523331824, 0.3000153484761401979, 0.3150161158999472133, 0.3300168833237542287, 0.3450176507475611887, 0.3600184181713682041, 0.3750191855951752196, 0.3900199530189822350, 0.4050207204427892504, 0.4200214878665962659, 0.4350222552904032813, 0.4500230227142102968, 0.4650237901380173122, 0.4800245575618242722, 0.4950253249856312876, 0.5100260924094383030, 0.5250268598332453740, 0.5400276272570523339, 0.5550283946808592939, 0.5700291621046663648, 0.5850299295284733248, 0.6000306969522803957, 0.6150314643760873556, 0.6300322317998944266, 0.6450329992237013865, 0.6600337666475084575, 0.6750345340713154174, 0.6900353014951223773, 0.7050360689189294483, 0.7200368363427364082, 0.7350376037665434792, 0.7500383711903504391, 0.7650391386141575101, 0.7800399060379644700, 0.7950406734617715410, 0.8100414408855785009, 0.8250422083093854608, 0.8400429757331925318, 0.8550437431569994917, 0.8700445105808065627, 0.8850452780046135226, 0.9000460454284205936, 0.9150468128522275535, 0.9300475802760346244, 0.9450483476998415844, 0.9600491151236485443, 0.9750498825474556153, 0.9900506499712625752, 1.000000000000000000 ),
 .UNSPECIFIED. ) 
 CURVE ( )  GEOMETRIC_REPRESENTATION_ITEM ( )  RATIONAL_B_SPLINE_CURVE ( ( 1.000000000000000000, 0.8660254037844387076, 1.000000000000000000, 0.8660254037844387076, 1.000000000000000000, 0.8660254037844387076, 1.000000000000000000, 0.8660254037844387076, 1.000000000000000000, 0.8660254037844387076, 1.000000000000000000, 0.8660254037844387076, 1.000000000000000000, 0.8660254037844387076, 1.000000000000000000, 0.8660254037844387076, 1.000000000000000000, 0.8660254037844387076, 1.000000000000000000, 0.8660254037844387076, 1.000000000000000000, 0.8660254037844387076, 1.000000000000000000, 0.8660254037844387076, 1.000000000000000000, 0.8660254037844387076, 1.000000000000000000, 0.8660254037844387076, 1.000000000000000000, 0.8660254037844387076, 1.000000000000000000, 0.8660254037844387076, 1.000000000000000000, 0.8660254037844387076, 1.000000000000000000, 0.8660254037844387076, 1.000000000000000000, 0.8660254037844387076, 1.000000000000000000, 0.8660254037844387076, 1.000000000000000000, 0.8660254037844387076, 1.000000000000000000, 0.8660254037844387076, 1.000000000000000000, 0.8660254037844387076, 1.000000000000000000, 0.8660254037844387076, 1.000000000000000000, 0.8660254037844387076, 1.000000000000000000, 0.8660254037844387076, 1.000000000000000000, 0.8660254037844387076, 1.000000000000000000, 0.8660254037844387076, 1.000000000000000000, 0.8660254037844387076, 1.000000000000000000, 0.8660254037844387076, 1.000000000000000000, 0.8660254037844387076, 1.000000000000000000, 0.8660254037844387076, 1.000000000000000000, 0.8660254037844387076, 1.000000000000000000, 0.8660254037844387076, 1.000000000000000000, 0.8660254037844387076, 1.000000000000000000, 0.8660254037844387076, 1.000000000000000000, 0.8660254037844387076, 1.000000000000000000, 0.8660254037844387076, 1.000000000000000000, 0.8660254037844387076, 1.000000000000000000, 0.8660254037844387076, 1.000000000000000000, 0.8660254037844387076, 1.000000000000000000, 0.8660254037844387076, 1.000000000000000000, 0.8660254037844387076, 1.000000000000000000, 0.8660254037844387076, 1.000000000000000000, 0.8660254037844387076, 1.000000000000000000, 0.8660254037844387076, 1.000000000000000000, 0.8660254037844387076, 1.000000000000000000, 0.8660254037844387076, 1.000000000000000000, 0.8660254037844387076, 1.000000000000000000, 0.8660254037844387076, 1.000000000000000000, 0.8660254037844387076, 1.000000000000000000, 0.8660254037844387076, 1.000000000000000000, 0.8660254037844387076, 1.000000000000000000, 0.8660254037844387076, 1.000000000000000000, 0.8660254037844387076, 1.000000000000000000, 0.8660254037844387076, 1.000000000000000000, 0.8660254037844387076, 1.000000000000000000, 0.8660254037844387076, 1.000000000000000000, 0.8660254037844387076, 1.000000000000000000, 0.8660254037844387076, 1.000000000000000000, 0.8660254037844387076, 1.000000000000000000, 0.8660254037844387076, 1.000000000000000000, 0.8660254037844387076, 1.000000000000000000, 0.8660254037844387076, 1.000000000000000000, 0.8660254037844387076, 1.000000000000000000, 0.8660254037844387076, 1.000000000000000000, 0.9111405360107182050, 0.9401542295229976531 ) ) 
 REPRESENTATION_ITEM ( '' )  );
#7435=CARTESIAN_POINT ( 'NONE',  ( 2.256430356250000546, -0.5156249993854828961, 1.302750673588579877 ) ) ;
#7443=CARTESIAN_POINT ( 'NONE',  ( 4.996790860652426159E-15, -1.462499999999999911, -2.500000000000000000 ) ) ;
#7466=CARTESIAN_POINT ( 'NONE',  ( 0.6698729810778112359, -4.632596189432333311, -2.499999999999996447 ) ) ;
#7467=CARTESIAN_POINT ( 'NONE',  ( 1.250000000000001110, -0.2999999999999999889, 2.165063509461096380 ) ) ;
#7472=EDGE_CURVE ( 'NONE', #5726, #2184, #8068, .T. ) ;
#7478=EDGE_CURVE ( 'NONE', #4703, #1808, #3328, .T. ) ;
#7483=CARTESIAN_POINT ( 'NONE',  ( -1.728529299398585906, -5.253648441416169490, -1.450401466387756244 ) ) ;
#7485=EDGE_CURVE ( 'NONE', #4596, #8813, #6522, .T. ) ;
#7490=CARTESIAN_POINT ( 'NONE',  ( -1.128215178125000273, -1.228124999385483029, -1.954126010382871259 ) ) ;
#7492=CARTESIAN_POINT ( 'NONE',  ( 6.123233995736727825E-17, -25.00000000000000000, 0.4999999999999968914 ) ) ;
#7495=DIRECTION ( 'NONE',  ( 0.000000000000000000, 0.000000000000000000, -1.000000000000000000 ) ) ;
#7497=ADVANCED_FACE ( 'NONE', ( #8241 ), #979, .T. ) ;
#7498=CARTESIAN_POINT ( 'NONE',  ( 0.000000000000000000, 0.000000000000000000, 0.000000000000000000 ) ) ;
#7501=EDGE_LOOP ( 'NONE', ( #2121, #2075, #9108, #5475 ) ) ;
#7508=ORIENTED_EDGE ( 'NONE', *, *, #7390, .F. ) ;
#7511=CARTESIAN_POINT ( 'NONE',  ( -3.000000000000000888, -15.00000000000000000, -1.732050807568877415 ) ) ;
#7516=CARTESIAN_POINT ( 'NONE',  ( -4.357666448243394824E-15, -2.137500000000000178, 2.500000000000000000 ) ) ;
#7518=CARTESIAN_POINT ( 'NONE',  ( -2.499999999999999556, -1.762499999999999734, 1.443375672974065882 ) ) ;
#7520=CARTESIAN_POINT ( 'NONE',  ( -4.357666448243394824E-15, -2.587499999999999467, 2.500000000000000000 ) ) ;
#7530=CARTESIAN_POINT ( 'NONE',  ( -2.256430356249999214, -0.5531249993854828739, 1.302750673588581876 ) ) ;
#7531=DIRECTION ( 'NONE',  ( 0.000000000000000000, 0.000000000000000000, -1.000000000000000000 ) ) ;
#7533=CARTESIAN_POINT ( 'NONE',  ( -2.500000000000000000, -1.781249998770965570, -1.443375672974064106 ) ) ;
#7534=VECTOR ( 'NONE', #2340, 1000.000000000000000 ) ;
#7540=CARTESIAN_POINT ( 'NONE',  ( -1.128215178124998497, -1.078124999385482674, 1.954126010382872147 ) ) ;
#7541=VERTEX_POINT ( 'NONE', #338 ) ;
#7546=DIRECTION ( 'NONE',  ( -2.406779422944247204E-17, 0.9949358851208914833, 0.1005116137503925117 ) ) ;
#7554=AXIS2_PLACEMENT_3D ( 'NONE', #4432, #352, #1035 ) ;
#7561=VERTEX_POINT ( 'NONE', #4124 ) ;
#7566=DIRECTION ( 'NONE',  ( 0.000000000000000000, 0.000000000000000000, -1.000000000000000000 ) ) ;
#7568=EDGE_LOOP ( 'NONE', ( #10365, #7923, #770, #721, #2973, #7995 ) ) ;
#7572=CARTESIAN_POINT ( 'NONE',  ( 2.500000000000000444, -1.612499999999999822, 1.443375672974063439 ) ) ;
#7573=SHAPE_DEFINITION_REPRESENTATION ( #8867, #9736 ) ;
#7575=CARTESIAN_POINT ( 'NONE',  ( 1.128215178125001161, -0.5531249993854828739, 1.954126010382870815 ) ) ;
#7577=CARTESIAN_POINT ( 'NONE',  ( -0.6698729810778069060, -0.9924038105676656896, -2.500000000000000000 ) ) ;
#7595=CARTESIAN_POINT ( 'NONE',  ( -2.256430356250000102, -1.640624999385482896, -1.302750673588580321 ) ) ;
#7598=LINE ( 'NONE', #8559, #6123 ) ;
#7604=EDGE_CURVE ( 'NONE', #7920, #1900, #2598, .T. ) ;
#7609=ORIENTED_EDGE ( 'NONE', *, *, #4381, .T. ) ;
#7616=CARTESIAN_POINT ( 'NONE',  ( 0.000000000000000000, -20.00000000000000000, 0.000000000000000000 ) ) ;
#7625=CARTESIAN_POINT ( 'NONE',  ( -1.767625397874844694E-16, -1.012499999999999956, -2.886751345948128655 ) ) ;
#7627=CARTESIAN_POINT ( 'NONE',  ( -9.703070624755296135E-15, -3.937500000000000888, 2.500000000000000444 ) ) ;
#7628=CARTESIAN_POINT ( 'NONE',  ( 1.128215178125001161, -2.803124999385482319, 1.954126010382870815 ) ) ;
#7633=MECHANICAL_DESIGN_GEOMETRIC_PRESENTATION_REPRESENTATION('',(#1947),#10335);
#7637=CARTESIAN_POINT ( 'NONE',  ( 4.786228327491940187E-16, -2.278124999385482852, 2.605501347177161087 ) ) ;
#7652=CARTESIAN_POINT ( 'NONE',  ( -1.595409442497313560E-16, -2.165624999385483029, -2.605501347177161087 ) ) ;
#7656=CARTESIAN_POINT ( 'NONE',  ( 2.500000000000000000, -0.6375000000000000666, -1.443375672974065438 ) ) ;
#7669=CARTESIAN_POINT ( 'NONE',  ( -2.256430356250000102, -0.5906249993854829627, 0.000000000000000000 ) ) ;
#7682=CARTESIAN_POINT ( 'NONE',  ( -2.499999999999999556, -2.212499999999999467, 1.443375672974065882 ) ) ;
#7686=CARTESIAN_POINT ( 'NONE',  ( -2.256430356249999214, -1.565624999385482718, 1.302750673588581876 ) ) ;
#7690=UNCERTAINTY_MEASURE_WITH_UNIT (LENGTH_MEASURE( 1.000000000000000082E-05 ), #1042, 'distance_accuracy_value', 'NONE');
#7691=CARTESIAN_POINT ( 'NONE',  ( 1.249999999999999334, -1.949999999999999956, -2.165063509461096825 ) ) ;
#7695=AXIS2_PLACEMENT_3D ( 'NONE', #7511, #2608, #7360 ) ;
#7697=CARTESIAN_POINT ( 'NONE',  ( -1.128215178124998497, -1.415624999385482807, 1.954126010382872147 ) ) ;
#7699=EDGE_LOOP ( 'NONE', ( #6110, #4621, #1501, #8543 ) ) ;
#7700=CARTESIAN_POINT ( 'NONE',  ( 2.256430356249999658, -0.3281249993854829516, -1.302750673588581432 ) ) ;
#7708=ORIENTED_EDGE ( 'NONE', *, *, #2294, .T. ) ;
#7710=CARTESIAN_POINT ( 'NONE',  ( -2.256430356250000102, -0.7406249993854829849, -1.302750673588580321 ) ) ;
#7714=CARTESIAN_POINT ( 'NONE',  ( -2.256430356250000102, -0.7031249993854828961, 0.000000000000000000 ) ) ;
#7718=CARTESIAN_POINT ( 'NONE',  ( -2.500000000000000000, -0.4312499987709658700, -1.443375672974064106 ) ) ;
#7724=CARTESIAN_POINT ( 'NONE',  ( -1.249999999999998224, -4.368749998770964815, 2.165063509461097713 ) ) ;
#7725=CARTESIAN_POINT ( 'NONE',  ( -2.256430356249999214, -2.353124999385482585, 1.302750673588581876 ) ) ;
#7738=CARTESIAN_POINT ( 'NONE',  ( -2.500000000000000000, -2.699999999999999734, 0.000000000000000000 ) ) ;
#7742=CARTESIAN_POINT ( 'NONE',  ( -2.256430356249999214, -2.465624999385482852, 1.302750673588581876 ) ) ;
#7746=AXIS2_PLACEMENT_3D ( 'NONE', #9264, #4561, #3782 ) ;
#7749=ADVANCED_FACE ( 'NONE', ( #3694 ), #3584, .T. ) ;
#7754=ORIENTED_EDGE ( 'NONE', *, *, #10299, .F. ) ;
#7755=CARTESIAN_POINT ( 'NONE',  ( 1.128215178124999607, -1.190624999385482941, -1.954126010382871259 ) ) ;
#7756=CARTESIAN_POINT ( 'NONE',  ( -2.256430356250000102, -0.1406249993854829794, 0.000000000000000000 ) ) ;
#7758=CARTESIAN_POINT ( 'NONE',  ( -0.6698729810778069060, -1.386153809338631415, -2.500000000000000000 ) ) ;
#7768=CARTESIAN_POINT ( 'NONE',  ( 2.256430356249999658, -4.490624999385483207, -1.302750673588581432 ) ) ;
#7773=CARTESIAN_POINT ( 'NONE',  ( -1.128215178124998497, -1.078124999385482674, 1.954126010382872147 ) ) ;
#7775=CARTESIAN_POINT ( 'NONE',  ( 1.249999999999999334, -0.5437499987709658589, -2.165063509461096825 ) ) ;
#7776=CIRCLE ( 'NONE', #8624, 2.500000000000000000 ) ;
#7780=CARTESIAN_POINT ( 'NONE',  ( -1.128215178125000273, -1.565624999385482941, -1.954126010382871259 ) ) ;
#7793=CARTESIAN_POINT ( 'NONE',  ( -1.249999999999998224, -4.424999999999998934, 2.165063509461097713 ) ) ;
#7796=CARTESIAN_POINT ( 'NONE',  ( -1.128215178125000273, -2.128124999385482496, -1.954126010382871259 ) ) ;
#7799=UNCERTAINTY_MEASURE_WITH_UNIT (LENGTH_MEASURE( 1.000000000000000082E-05 ), #6798, 'distance_accuracy_value', 'NONE');
#7806=CARTESIAN_POINT ( 'NONE',  ( 2.256430356250000102, -1.715624999385482852, -2.763330213280484622E-16 ) ) ;
#7810=CARTESIAN_POINT ( 'NONE',  ( 2.256430356249999658, -1.228124999385483029, -1.302750673588581432 ) ) ;
#7815=CARTESIAN_POINT ( 'NONE',  ( -4.357666448243394824E-15, -2.981249998770965526, 2.500000000000000000 ) ) ;
#7822=CARTESIAN_POINT ( 'NONE',  ( 2.256430356250000102, -4.528124999385481964, -2.763330213280484622E-16 ) ) ;
#7826=CARTESIAN_POINT ( 'NONE',  ( 1.250000000000001110, -0.2999999999999999889, 2.165063509461096380 ) ) ;
#7827=ADVANCED_FACE ( 'NONE', ( #6769 ), #2707, .T. ) ;
#7828=CARTESIAN_POINT ( 'NONE',  ( 4.786228327491940187E-16, -1.490624999385482541, 2.605501347177161087 ) ) ;
#7830=FACE_OUTER_BOUND ( 'NONE', #1177, .T. ) ;
#7832=CARTESIAN_POINT ( 'NONE',  ( -1.767625397874844694E-16, -1.406249998770965570, -2.886751345948128655 ) ) ;
#7835=ORIENTED_EDGE ( 'NONE', *, *, #6832, .T. ) ;
#7836=CARTESIAN_POINT ( 'NONE',  ( 3.061616997868383141E-16, 0.000000000000000000, 2.500000000000000000 ) ) ;
#7837=CARTESIAN_POINT ( 'NONE',  ( 2.256430356250000102, -1.265624999385482896, -2.763330213280484622E-16 ) ) ;
#7841=ADVANCED_FACE ( 'NONE', ( #8763 ), #7975, .T. ) ;
#7850=CARTESIAN_POINT ( 'NONE',  ( -1.128215178124998497, -1.078124999385482674, 1.954126010382872147 ) ) ;
#7853=( BOUNDED_CURVE ( )  B_SPLINE_CURVE ( 2, ( #455, #3651, #6829, #6214, #9294, #3814, #6997, #5328, #1344 ),
 .UNSPECIFIED., .F., .T. ) 
 B_SPLINE_CURVE_WITH_KNOTS ( ( 3, 2, 2, 2, 3 ),
 ( 0.06250000000000000000, 0.06944444444444444753, 0.08333333333333332871, 0.09722222222222222376, 0.1041666666666666713 ),
 .UNSPECIFIED. ) 
 CURVE ( )  GEOMETRIC_REPRESENTATION_ITEM ( )  RATIONAL_B_SPLINE_CURVE ( ( 0.9330127018922194093, 0.9330127018922194093, 1.000000000000000000, 0.8660254037844387076, 1.000000000000000000, 0.8660254037844387076, 1.000000000000000000, 0.9330127018922192983, 0.9330127018922194093 ) ) 
 REPRESENTATION_ITEM ( '' )  );
#7855=CARTESIAN_POINT ( 'NONE',  ( -2.500000000000000000, -3.093749998770965348, 0.000000000000000000 ) ) ;
#7857=EDGE_CURVE ( 'NONE', #5955, #9728, #1799, .T. ) ;
#7860=CARTESIAN_POINT ( 'NONE',  ( 1.128215178125001161, -2.240624999385482763, 1.954126010382870815 ) ) ;
#7863=CARTESIAN_POINT ( 'NONE',  ( -2.256430356250000102, -1.978124999385482807, -1.302750673588580321 ) ) ;
#7871=CARTESIAN_POINT ( 'NONE',  ( 2.256430356249999658, -3.140624999385482674, -1.302750673588581432 ) ) ;
#7872=VERTEX_POINT ( 'NONE', #1863 ) ;
#7874=DIRECTION ( 'NONE',  ( 0.000000000000000000, -1.000000000000000000, 0.000000000000000000 ) ) ;
#7875=CARTESIAN_POINT ( 'NONE',  ( 1.128215178124999607, -2.653124999385482408, -1.954126010382871259 ) ) ;
#7878=EDGE_CURVE ( 'NONE', #5471, #7399, #2642, .T. ) ;
#7881=CARTESIAN_POINT ( 'NONE',  ( 1.250000000000001110, -1.593749998770965792, 2.165063509461096380 ) ) ;
#7886=CARTESIAN_POINT ( 'NONE',  ( 0.6698729810778075722, -4.367403810567665801, 2.499999999999999556 ) ) ;
#7887=CARTESIAN_POINT ( 'NONE',  ( 1.128215178125001161, -2.240624999385482763, 1.954126010382870815 ) ) ;
#7899=CARTESIAN_POINT ( 'NONE',  ( 2.500000000000000000, -4.274999999999999467, -3.061616997868383141E-16 ) ) ;
#7902=CARTESIAN_POINT ( 'NONE',  ( -1.595409442497313560E-16, -4.865624999385482319, -2.605501347177161087 ) ) ;
#7905=CIRCLE ( 'NONE', #1712, 0.4999999999999968914 ) ;
#7910=CARTESIAN_POINT ( 'NONE',  ( -1.128215178125000273, -3.815624999385482941, -1.954126010382871259 ) ) ;
#7913=CARTESIAN_POINT ( 'NONE',  ( -2.256430356249999214, -1.453124999385482896, 1.302750673588581876 ) ) ;
#7920=VERTEX_POINT ( 'NONE', #6734 ) ;
#7921=LINE ( 'NONE', #7332, #5315 ) ;
#7923=ORIENTED_EDGE ( 'NONE', *, *, #4748, .T. ) ;
#7924=ORIENTED_EDGE ( 'NONE', *, *, #4198, .F. ) ;
#7925=CARTESIAN_POINT ( 'NONE',  ( -2.256430356250000102, -5.203124999385482674, 0.000000000000000000 ) ) ;
#7930=CARTESIAN_POINT ( 'NONE',  ( -2.256430356250000102, -2.503124999385482496, 0.000000000000000000 ) ) ;
#7936=CARTESIAN_POINT ( 'NONE',  ( -1.250000000000000222, -3.168749998770965526, -2.165063509461096825 ) ) ;
#7938=CARTESIAN_POINT ( 'NONE',  ( 2.500000000000000000, -1.068749998770965881, -3.061616997868383141E-16 ) ) ;
#7939=CARTESIAN_POINT ( 'NONE',  ( -2.500000000000000000, -3.149999999999999467, 0.000000000000000000 ) ) ;
#7942=CARTESIAN_POINT ( 'NONE',  ( -1.128215178124998497, -3.215624999385482408, 1.954126010382872147 ) ) ;
#7953=CARTESIAN_POINT ( 'NONE',  ( 5.302876193624534821E-16, -4.837500000000000355, 2.886751345948128655 ) ) ;
#7955=CARTESIAN_POINT ( 'NONE',  ( -2.256430356250000102, -4.303124999385482319, 0.000000000000000000 ) ) ;
#7963=CARTESIAN_POINT ( 'NONE',  ( -2.256430356250000102, -3.778124999385482408, -1.302750673588580321 ) ) ;
#7966=ORIENTED_EDGE ( 'NONE', *, *, #6082, .T. ) ;
#7967=CARTESIAN_POINT ( 'NONE',  ( 2.256430356250000102, -1.265624999385482896, -2.763330213280484622E-16 ) ) ;
#7969=FACE_OUTER_BOUND ( 'NONE', #7568, .T. ) ;
#7971=CARTESIAN_POINT ( 'NONE',  ( -2.256430356250000102, -0.2531249993854829405, 0.000000000000000000 ) ) ;
#7975=CYLINDRICAL_SURFACE ( 'NONE', #9824, 2.500000000000000000 ) ;
#7980=DIRECTION ( 'NONE',  ( -0.8660254037844385966, -0.000000000000000000, -0.5000000000000001110 ) ) ;
#7981=VECTOR ( 'NONE', #5698, 1000.000000000000000 ) ;
#7983=CARTESIAN_POINT ( 'NONE',  ( -2.256430356250000102, -3.403124999385482408, 0.000000000000000000 ) ) ;
#7988=CARTESIAN_POINT ( 'NONE',  ( 1.250000000000001110, -2.943749998770965437, 2.165063509461096380 ) ) ;
#7992=CARTESIAN_POINT ( 'NONE',  ( 0.000000000000000000, 0.000000000000000000, 0.000000000000000000 ) ) ;
#7994=CARTESIAN_POINT ( 'NONE',  ( -1.595409442497313560E-16, -2.953124999385482674, -2.605501347177161087 ) ) ;
#7995=ORIENTED_EDGE ( 'NONE', *, *, #3140, .F. ) ;
#7996=CARTESIAN_POINT ( 'NONE',  ( 3.000000000000000000, -15.00000000000000000, -1.732050807568876749 ) ) ;
#7999=CARTESIAN_POINT ( 'NONE',  ( 0.6698729810778075722, -2.061153809338631238, 2.499999999999999556 ) ) ;
#8000=LINE ( 'NONE', #5648, #7981 ) ;
#8004=CARTESIAN_POINT ( 'NONE',  ( -2.500000000000000000, -4.049999999999999822, 0.000000000000000000 ) ) ;
#8007=CARTESIAN_POINT ( 'NONE',  ( 2.256430356250000546, -3.665624999385482141, 1.302750673588579877 ) ) ;
#8017=CARTESIAN_POINT ( 'NONE',  ( -1.128215178125000273, -2.915624999385482585, -1.954126010382871259 ) ) ;
#8018=CARTESIAN_POINT ( 'NONE',  ( 0.6698729810778063509, -2.382596189432333755, -2.500000000000000000 ) ) ;
#8020=CARTESIAN_POINT ( 'NONE',  ( 4.786228327491941173E-16, -1.828124999385482896, 2.605501347177161087 ) ) ;
#8023=DIRECTION ( 'NONE',  ( 0.000000000000000000, 0.000000000000000000, -1.000000000000000000 ) ) ;
#8031=CARTESIAN_POINT ( 'NONE',  ( 2.500000000000000000, -4.181249998770965703, -1.443375672974065438 ) ) ;
#8034=CARTESIAN_POINT ( 'NONE',  ( -2.256430356249998770, -4.715624999385481964, 1.302750673588581876 ) ) ;
#8038=CARTESIAN_POINT ( 'NONE',  ( 1.249999999999999334, -2.343749998770965792, -2.165063509461096825 ) ) ;
#8043=CARTESIAN_POINT ( 'NONE',  ( 2.256430356249999658, -3.028124999385482852, -1.302750673588581432 ) ) ;
#8050=VERTEX_POINT ( 'NONE', #9363 ) ;
#8054=CARTESIAN_POINT ( 'NONE',  ( 2.256430356250000546, -3.215624999385482408, 1.302750673588579877 ) ) ;
#8060=CYLINDRICAL_SURFACE ( 'NONE', #6406, 2.500000000000000000 ) ;
#8063=CARTESIAN_POINT ( 'NONE',  ( -1.128215178125000273, -3.365624999385482763, -1.954126010382871259 ) ) ;
#8067=CARTESIAN_POINT ( 'NONE',  ( 4.786228327491941173E-16, -3.628124999385482941, 2.605501347177161087 ) ) ;
#8068=( BOUNDED_CURVE ( )  B_SPLINE_CURVE ( 2, ( #6275, #10361, #3192, #8785, #6479, #1610, #4804, #7999, #9668 ),
 .UNSPECIFIED., .F., .F. ) 
 B_SPLINE_CURVE_WITH_KNOTS ( ( 3, 2, 2, 2, 3 ),
 ( 0.2708333333333333703, 0.2777777777777777901, 0.2916666666666666852, 0.3055555555555555802, 0.3125000000000000000 ),
 .UNSPECIFIED. ) 
 CURVE ( )  GEOMETRIC_REPRESENTATION_ITEM ( )  RATIONAL_B_SPLINE_CURVE ( ( 0.9330127018922194093, 0.9330127018922196314, 1.000000000000000000, 0.8660254037844387076, 1.000000000000000000, 0.8660254037844387076, 1.000000000000000000, 0.9330127018922194093, 0.9330127018922194093 ) ) 
 REPRESENTATION_ITEM ( '' )  );
#8073=AXIS2_PLACEMENT_3D ( 'NONE', #10179, #4628, #5473 ) ;
#8074=EDGE_CURVE ( 'NONE', #5471, #4614, #8000, .T. ) ;
#8077=ORIENTED_EDGE ( 'NONE', *, *, #6253, .T. ) ;
#8078=DIRECTION ( 'NONE',  ( 0.000000000000000000, 0.000000000000000000, -1.000000000000000000 ) ) ;
#8086=CARTESIAN_POINT ( 'NONE',  ( -1.595409442497313560E-16, -4.865624999385482319, -2.605501347177161087 ) ) ;
#8091=CARTESIAN_POINT ( 'NONE',  ( -1.250000000000000222, -4.068749998770965881, -2.165063509461096825 ) ) ;
#8095=CARTESIAN_POINT ( 'NONE',  ( -3.061616997868383634E-16, -20.00000000000000000, 2.500000000000000444 ) ) ;
#8097=CARTESIAN_POINT ( 'NONE',  ( 2.256430356250000102, -3.965624999385482408, -2.763330213280484622E-16 ) ) ;
#8108=CARTESIAN_POINT ( 'NONE',  ( 2.256430356249999658, -0.3281249993854829516, -1.302750673588581432 ) ) ;
#8111=FACE_OUTER_BOUND ( 'NONE', #4418, .T. ) ;
#8115=CARTESIAN_POINT ( 'NONE',  ( 4.786228327491940187E-16, -3.628124999385482941, 2.605501347177161087 ) ) ;
#8117=CARTESIAN_POINT ( 'NONE',  ( -1.214319963873739860, -5.167334288697576383, -2.063219373018434943 ) ) ;
#8123=FACE_OUTER_BOUND ( 'NONE', #4375, .T. ) ;
#8129=ORIENTED_EDGE ( 'NONE', *, *, #9605, .T. ) ;
#8130=DIRECTION ( 'NONE',  ( 0.000000000000000000, -1.000000000000000000, 0.000000000000000000 ) ) ;
#8133=CARTESIAN_POINT ( 'NONE',  ( 1.128215178124999607, -4.453124999385482674, -1.954126010382871259 ) ) ;
#8136=AXIS2_PLACEMENT_3D ( 'NONE', #2589, #4941, #9802 ) ;
#8138=CARTESIAN_POINT ( 'NONE',  ( -2.500000000000000000, -3.543749998770965526, 0.000000000000000000 ) ) ;
#8146=CARTESIAN_POINT ( 'NONE',  ( 2.256430356250000546, -4.903124999385481964, 1.302750673588579877 ) ) ;
#8156=PLANE ( 'NONE',  #2274 ) ;
#8162=ORIENTED_EDGE ( 'NONE', *, *, #3465, .F. ) ;
#8163=CARTESIAN_POINT ( 'NONE',  ( 2.256430356250000102, -4.415624999385482141, -2.763330213280484622E-16 ) ) ;
#8170=CARTESIAN_POINT ( 'NONE',  ( -2.500000000000000000, -1.387499999999999734, -1.443375672974064106 ) ) ;
#8178=CARTESIAN_POINT ( 'NONE',  ( 2.256430356249999658, -3.590624999385482408, -1.302750673588581432 ) ) ;
#8184=CARTESIAN_POINT ( 'NONE',  ( -1.128215178125000273, -0.3281249993854828961, -1.954126010382871259 ) ) ;
#8193=CARTESIAN_POINT ( 'NONE',  ( 2.500000000000000000, -1.537500000000000089, -1.443375672974065438 ) ) ;
#8207=CARTESIAN_POINT ( 'NONE',  ( -2.500000000000000000, -2.250000000000000000, 0.000000000000000000 ) ) ;
#8209=CARTESIAN_POINT ( 'NONE',  ( 2.256430356250000546, -3.553124999385482763, 1.302750673588579877 ) ) ;
#8210=SURFACE_SIDE_STYLE ('',( #4964 ) ) ;
#8215=CIRCLE ( 'NONE', #711, 0.4999999999999968914 ) ;
#8216=CARTESIAN_POINT ( 'NONE',  ( 4.996790860652426159E-15, -1.462499999999999911, -2.500000000000000000 ) ) ;
#8223=ADVANCED_FACE ( 'NONE', ( #9713 ), #192, .T. ) ;
#8231=CARTESIAN_POINT ( 'NONE',  ( -2.500000000000000000, -5.367390388364559506, -0.9099190197072017927 ) ) ;
#8241=FACE_OUTER_BOUND ( 'NONE', #2086, .T. ) ;
#8242=EDGE_CURVE ( 'NONE', #2028, #9475, #4995, .T. ) ;
#8250=DIRECTION ( 'NONE',  ( 0.000000000000000000, 0.000000000000000000, -1.000000000000000000 ) ) ;
#8252=EDGE_CURVE ( 'NONE', #3336, #1163, #920, .T. ) ;
#8260=CARTESIAN_POINT ( 'NONE',  ( -2.500000000000000000, -4.931249998770965703, -1.443375672974064106 ) ) ;
#8262=CARTESIAN_POINT ( 'NONE',  ( 1.128215178124999607, -4.790624999385483029, -1.954126010382871259 ) ) ;
#8275=DIRECTION ( 'NONE',  ( -0.000000000000000000, 1.000000000000000000, -0.000000000000000000 ) ) ;
#8276=CARTESIAN_POINT ( 'NONE',  ( -2.256430356250000102, -5.203124999385482674, 0.000000000000000000 ) ) ;
#8277=CARTESIAN_POINT ( 'NONE',  ( 9.877377282685029372E-16, -4.387499999999999289, 2.500000000000000000 ) ) ;
#8282=CARTESIAN_POINT ( 'NONE',  ( -1.249999999999998224, -3.468749998770965348, 2.165063509461097713 ) ) ;
#8286=CARTESIAN_POINT ( 'NONE',  ( -3.000000000000000888, -15.00000000000000000, -1.732050807568877415 ) ) ;
#8287=CARTESIAN_POINT ( 'NONE',  ( 3.061616997868383141E-16, 0.000000000000000000, 2.500000000000000000 ) ) ;
#8299=CARTESIAN_POINT ( 'NONE',  ( -0.6698729810778020211, -4.592403810567665445, -2.500000000000002665 ) ) ;
#8304=CARTESIAN_POINT ( 'NONE',  ( 2.500000000000000000, -4.631249998770966769, -1.443375672974065438 ) ) ;
#8305=LINE ( 'NONE', #5210, #211 ) ;
#8309=CARTESIAN_POINT ( 'NONE',  ( -1.249999999999998224, -4.818749998770964993, 2.165063509461097713 ) ) ;
#8311=CARTESIAN_POINT ( 'NONE',  ( -2.500000000000000000, -1.349999999999999867, 0.000000000000000000 ) ) ;
#8314=DIRECTION ( 'NONE',  ( -0.000000000000000000, -0.000000000000000000, 1.000000000000000000 ) ) ;
#8322=DIRECTION ( 'NONE',  ( 0.000000000000000000, -1.000000000000000000, 0.000000000000000000 ) ) ;
#8326=CARTESIAN_POINT ( 'NONE',  ( -0.6698729810778105698, -5.251346188203299903, 2.499999999999997780 ) ) ;
#8327=CARTESIAN_POINT ( 'NONE',  ( 1.128215178125001161, -0.4406249993854829405, 1.954126010382870815 ) ) ;
#8331=LINE ( 'NONE', #273, #5450 ) ;
#8333=ORIENTED_EDGE ( 'NONE', *, *, #9948, .T. ) ;
#8335=CARTESIAN_POINT ( 'NONE',  ( 2.256430356249999658, -1.790624999385482807, -1.302750673588581432 ) ) ;
#8344=CARTESIAN_POINT ( 'NONE',  ( 1.034219503716432668E-14, -3.656249998770965792, -2.500000000000000000 ) ) ;
#8350=EDGE_CURVE ( 'NONE', #2028, #10197, #5912, .T. ) ;
#8353=EDGE_LOOP ( 'NONE', ( #230, #3907, #8613 ) ) ;
#8360=DIRECTION ( 'NONE',  ( 0.000000000000000000, -1.000000000000000000, 0.000000000000000000 ) ) ;
#8361=CARTESIAN_POINT ( 'NONE',  ( -2.500000000000000000, -4.893749998770965171, 0.000000000000000000 ) ) ;
#8364=CARTESIAN_POINT ( 'NONE',  ( -1.250000000000000222, -1.424999999999999822, -2.165063509461096825 ) ) ;
#8368=CARTESIAN_POINT ( 'NONE',  ( 2.256430356250000102, -0.4781249993854829183, -2.763330213280484622E-16 ) ) ;
#8379=CARTESIAN_POINT ( 'NONE',  ( 2.256430356249999658, -0.7781249993854829627, -1.302750673588581432 ) ) ;
#8381=ADVANCED_FACE ( 'NONE', ( #391 ), #3807, .T. ) ;
#8386=EDGE_LOOP ( 'NONE', ( #6744, #8933 ) ) ;
#8388=CARTESIAN_POINT ( 'NONE',  ( 2.256430356250000546, -1.865624999385482985, 1.302750673588579877 ) ) ;
#8395=DIRECTION ( 'NONE',  ( 0.000000000000000000, 0.000000000000000000, -1.000000000000000000 ) ) ;
#8403=DIRECTION ( 'NONE',  ( -0.08704561088320925122, 0.9949358851208914833, 0.05025580687519626277 ) ) ;
#8404=DIRECTION ( 'NONE',  ( 0.8660254037844385966, -0.000000000000000000, -0.5000000000000000000 ) ) ;
#8408=CARTESIAN_POINT ( 'NONE',  ( -2.500000000000000000, -3.993749998770965703, 0.000000000000000000 ) ) ;
#8409=DIRECTION ( 'NONE',  ( 0.000000000000000000, 0.000000000000000000, -1.000000000000000000 ) ) ;
#8416=CARTESIAN_POINT ( 'NONE',  ( 1.249999999999999334, -2.399999999999999911, -2.165063509461096825 ) ) ;
#8418=FACE_OUTER_BOUND ( 'NONE', #10106, .T. ) ;
#8419=CARTESIAN_POINT ( 'NONE',  ( 2.256430356250000102, -2.728124999385482585, -2.763330213280484622E-16 ) ) ;
#8429=CARTESIAN_POINT ( 'NONE',  ( -1.128215178124998497, -1.865624999385482763, 1.954126010382872147 ) ) ;
#8430=CARTESIAN_POINT ( 'NONE',  ( -2.256430356250000102, -0.2531249993854829405, 0.000000000000000000 ) ) ;
#8432=CARTESIAN_POINT ( 'NONE',  ( 4.786228327491941173E-16, -0.9281249993854827629, 2.605501347177161087 ) ) ;
#8438=ORIENTED_EDGE ( 'NONE', *, *, #1823, .T. ) ;
#8441=CARTESIAN_POINT ( 'NONE',  ( -1.128215178125000273, -2.578124999385482674, -1.954126010382871259 ) ) ;
#8442=ORIENTED_EDGE ( 'NONE', *, *, #6647, .F. ) ;
#8446=AXIS2_PLACEMENT_3D ( 'NONE', #4957, #1911, #1134 ) ;
#8447=CARTESIAN_POINT ( 'NONE',  ( 1.034219503716432668E-14, -5.006249998770964993, -2.500000000000000000 ) ) ;
#8458=CARTESIAN_POINT ( 'NONE',  ( 2.256430356250000102, -2.615624999385482763, -2.763330213280484622E-16 ) ) ;
#8466=CARTESIAN_POINT ( 'NONE',  ( -2.500000000000000000, -0.4874999999999999889, -1.443375672974064106 ) ) ;
#8467=EDGE_LOOP ( 'NONE', ( #6908, #7208, #1983, #1226 ) ) ;
#8472=CARTESIAN_POINT ( 'NONE',  ( -2.500000000000000000, -0.9000000000000000222, 0.000000000000000000 ) ) ;
#8475=DIRECTION ( 'NONE',  ( -0.6427814120798343023, 4.154457043096084790E-06, 0.7660496434744911154 ) ) ;
#8476=CARTESIAN_POINT ( 'NONE',  ( 2.256430356250000546, -0.9656249993854827407, 1.302750673588579877 ) ) ;
#8485=CARTESIAN_POINT ( 'NONE',  ( 2.256430356250000546, -2.203124999385482674, 1.302750673588579877 ) ) ;
#8486=CARTESIAN_POINT ( 'NONE',  ( 1.034219503716432668E-14, -4.162500000000000533, -2.500000000000000000 ) ) ;
#8497=DIRECTION ( 'NONE',  ( 0.4980973490458731057, -0.08715574274765838791, -0.8627299156628207566 ) ) ;
#8498=CARTESIAN_POINT ( 'NONE',  ( -1.128215178124998497, -2.878124999385482496, 1.954126010382872147 ) ) ;
#8500=AXIS2_PLACEMENT_3D ( 'NONE', #1815, #6679, #5109 ) ;
#8503=DIRECTION ( 'NONE',  ( 0.000000000000000000, -1.000000000000000000, 0.000000000000000000 ) ) ;
#8504=CARTESIAN_POINT ( 'NONE',  ( 1.128215178125001161, -1.453124999385482896, 1.954126010382870815 ) ) ;
#8508=CARTESIAN_POINT ( 'NONE',  ( 1.250000000000001110, -2.999999999999999556, 2.165063509461096380 ) ) ;
#8510=EDGE_CURVE ( 'NONE', #4631, #2830, #6645, .T. ) ;
#8512=CARTESIAN_POINT ( 'NONE',  ( 0.6698729810778112359, -4.182596189432334022, -2.499999999999996447 ) ) ;
#8513=CARTESIAN_POINT ( 'NONE',  ( -1.128215178125000273, -2.015624999385483118, -1.954126010382871259 ) ) ;
#8521=( BOUNDED_CURVE ( )  B_SPLINE_CURVE ( 2, ( #3346, #4332, #8309, #357, #8361, #8260, #5957, #5059, #4962 ),
 .UNSPECIFIED., .F., .T. ) 
 B_SPLINE_CURVE_WITH_KNOTS ( ( 3, 2, 2, 2, 3 ),
 ( 0.8125000000000000000, 0.8194444444444444198, 0.8333333333333333703, 0.8472222222222222099, 0.8541666666666667407 ),
 .UNSPECIFIED. ) 
 CURVE ( )  GEOMETRIC_REPRESENTATION_ITEM ( )  RATIONAL_B_SPLINE_CURVE ( ( 0.9330127018922194093, 0.9330127018922194093, 1.000000000000000000, 0.8660254037844387076, 1.000000000000000000, 0.8660254037844387076, 1.000000000000000000, 0.9330127018922187432, 0.9330127018922192983 ) ) 
 REPRESENTATION_ITEM ( '' )  );
#8523=ORIENTED_EDGE ( 'NONE', *, *, #9416, .T. ) ;
#8528=CARTESIAN_POINT ( 'NONE',  ( -1.767625397874844694E-16, -1.912499999999999867, -2.886751345948128655 ) ) ;
#8531=CARTESIAN_POINT ( 'NONE',  ( 2.256430356250000102, -1.378124999385482941, -2.763330213280484622E-16 ) ) ;
#8539=VECTOR ( 'NONE', #9093, 1000.000000000000000 ) ;
#8541=CARTESIAN_POINT ( 'NONE',  ( -2.256430356250000102, -2.390624999385482674, 0.000000000000000000 ) ) ;
#8543=ORIENTED_EDGE ( 'NONE', *, *, #3832, .T. ) ;
#8554=VERTEX_POINT ( 'NONE', #7096 ) ;
#8555=CARTESIAN_POINT ( 'NONE',  ( -1.128215178124998497, -1.978124999385482807, 1.954126010382872147 ) ) ;
#8559=CARTESIAN_POINT ( 'NONE',  ( -3.000000000000000888, -15.00000000000000000, -1.732050807568877415 ) ) ;
#8561=CARTESIAN_POINT ( 'NONE',  ( 4.786228327491940187E-16, -2.390624999385482230, 2.605501347177161087 ) ) ;
#8563=CARTESIAN_POINT ( 'NONE',  ( -2.500000000000000000, -1.800000000000000044, 0.000000000000000000 ) ) ;
#8565=ORIENTED_EDGE ( 'NONE', *, *, #5503, .T. ) ;
#8569=ORIENTED_EDGE ( 'NONE', *, *, #8887, .T. ) ;
#8570=CARTESIAN_POINT ( 'NONE',  ( 1.250000000000001110, -1.199999999999999956, 2.165063509461096380 ) ) ;
#8572=CARTESIAN_POINT ( 'NONE',  ( 2.256430356250000546, -0.4031249993854829627, 1.302750673588579877 ) ) ;
#8574=EDGE_LOOP ( 'NONE', ( #4101, #2800, #7377, #4460 ) ) ;
#8578=CARTESIAN_POINT ( 'NONE',  ( 4.996790860652426159E-15, -1.912499999999999867, -2.500000000000000000 ) ) ;
#8587=CARTESIAN_POINT ( 'NONE',  ( -2.500000000000000000, -3.187499999999999556, -1.443375672974064106 ) ) ;
#8590=CARTESIAN_POINT ( 'NONE',  ( -1.128215178125000273, -1.678124999385482763, -1.954126010382871259 ) ) ;
#8598=ADVANCED_FACE ( 'NONE', ( #138 ), #280, .F. ) ;
#8601=CARTESIAN_POINT ( 'NONE',  ( 1.128215178124999607, -0.7406249993854829849, -1.954126010382871259 ) ) ;
#8603=VERTEX_POINT ( 'NONE', #7492 ) ;
#8604=CARTESIAN_POINT ( 'NONE',  ( 1.128215178125001161, -2.240624999385482763, 1.954126010382870815 ) ) ;
#8612=CARTESIAN_POINT ( 'NONE',  ( 2.256430356250000102, -3.178124999385482319, -2.763330213280484622E-16 ) ) ;
#8613=ORIENTED_EDGE ( 'NONE', *, *, #9416, .F. ) ;
#8618=CARTESIAN_POINT ( 'NONE',  ( -1.595409442497313560E-16, -0.8156249993854828295, -2.605501347177161087 ) ) ;
#8620=EDGE_CURVE ( 'NONE', #4631, #4436, #3473, .T. ) ;
#8622=CARTESIAN_POINT ( 'NONE',  ( -1.767625397874844694E-16, -2.306249998770966148, -2.886751345948128655 ) ) ;
#8623=ORIENTED_EDGE ( 'NONE', *, *, #6274, .T. ) ;
#8624=AXIS2_PLACEMENT_3D ( 'NONE', #4129, #5049, #8250 ) ;
#8629=CARTESIAN_POINT ( 'NONE',  ( -2.256430356249999214, -0.5531249993854828739, 1.302750673588581876 ) ) ;
#8636=CARTESIAN_POINT ( 'NONE',  ( -1.249999999999998224, -3.468749998770965348, 2.165063509461097713 ) ) ;
#8637=VERTEX_POINT ( 'NONE', #6515 ) ;
#8641=LINE ( 'NONE', #8842, #8756 ) ;
#8643=CARTESIAN_POINT ( 'NONE',  ( 2.256430356249999658, -1.340624999385482852, -1.302750673588581432 ) ) ;
#8652=CARTESIAN_POINT ( 'NONE',  ( 2.256430356250000102, -0.3656249993854829294, -2.763330213280484622E-16 ) ) ;
#8655=CARTESIAN_POINT ( 'NONE',  ( 2.256430356250000102, -1.715624999385482852, -2.763330213280484622E-16 ) ) ;
#8657=ADVANCED_FACE ( 'NONE', ( #3368 ), #923, .T. ) ;
#8666=CARTESIAN_POINT ( 'NONE',  ( -2.256430356250000102, -4.790624999385483029, -1.302750673588580321 ) ) ;
#8671=CARTESIAN_POINT ( 'NONE',  ( 1.128215178125001161, -1.903124999385482852, 1.954126010382870815 ) ) ;
#8675=CARTESIAN_POINT ( 'NONE',  ( 2.500000000000000444, -2.006249998770965437, 1.443375672974063439 ) ) ;
#8676=CARTESIAN_POINT ( 'NONE',  ( 9.877377282685029372E-16, -1.181249998770965703, 2.500000000000000000 ) ) ;
#8679=CARTESIAN_POINT ( 'NONE',  ( 2.500000000000000000, -4.237499999999999822, -1.443375672974065438 ) ) ;
#8680=CARTESIAN_POINT ( 'NONE',  ( 4.786228327491941173E-16, -0.4781249993854829183, 2.605501347177161087 ) ) ;
#8685=CARTESIAN_POINT ( 'NONE',  ( -1.728530063377412329, -5.141148402510967941, -1.450400555903694766 ) ) ;
#8687=ORIENTED_EDGE ( 'NONE', *, *, #4224, .T. ) ;
#8692=CARTESIAN_POINT ( 'NONE',  ( -1.767625397874844694E-16, -4.612499999999998934, -2.886751345948128655 ) ) ;
#8695=CARTESIAN_POINT ( 'NONE',  ( 2.256430356249999658, -4.490624999385483207, -1.302750673588581432 ) ) ;
#8699=LINE ( 'NONE', #1637, #6326 ) ;
#8703=CARTESIAN_POINT ( 'NONE',  ( 1.128215178125001161, -2.690624999385482941, 1.954126010382870815 ) ) ;
#8708=CARTESIAN_POINT ( 'NONE',  ( 4.786228327491941173E-16, -2.278124999385482852, 2.605501347177161087 ) ) ;
#8712=CARTESIAN_POINT ( 'NONE',  ( -2.562556682370380035, -20.00000000000000000, 1.479492790380213751 ) ) ;
#8713=PRODUCT_DEFINITION ( 'UNKNOWN', '', #3812, #7062 ) ;
#8714=CYLINDRICAL_SURFACE ( 'NONE', #3472, 2.500000000000000000 ) ;
#8717=CARTESIAN_POINT ( 'NONE',  ( -1.128215178124998497, -5.128124999385482496, 1.954126010382872147 ) ) ;
#8722=CARTESIAN_POINT ( 'NONE',  ( 4.786228327491940187E-16, -0.5906249993854828517, 2.605501347177161087 ) ) ;
#8727=CARTESIAN_POINT ( 'NONE',  ( 1.249999999999999334, -1.893749998770965837, -2.165063509461096825 ) ) ;
#8730=CARTESIAN_POINT ( 'NONE',  ( 9.877377282685029372E-16, -3.037499999999999201, 2.500000000000000000 ) ) ;
#8732=CARTESIAN_POINT ( 'NONE',  ( -2.256430356250000102, -4.190624999385482496, 0.000000000000000000 ) ) ;
#8733=CONICAL_SURFACE ( 'NONE', #9881, 2.500000000000000444, 0.08726646259971666819 ) ;
#8741=CARTESIAN_POINT ( 'NONE',  ( -1.767625397874844694E-16, -3.262499999999999289, -2.886751345948128655 ) ) ;
#8743=CARTESIAN_POINT ( 'NONE',  ( 4.786228327491941173E-16, -3.290624999385482585, 2.605501347177161087 ) ) ;
#8750=FACE_OUTER_BOUND ( 'NONE', #149, .T. ) ;
#8751=CARTESIAN_POINT ( 'NONE',  ( 2.256430356250000102, -3.965624999385482408, -2.763330213280484622E-16 ) ) ;
#8753=CARTESIAN_POINT ( 'NONE',  ( -2.256430356250000102, -2.390624999385482674, 0.000000000000000000 ) ) ;
#8756=VECTOR ( 'NONE', #4173, 1000.000000000000000 ) ;
#8758=CARTESIAN_POINT ( 'NONE',  ( -3.486133158594716510E-16, -4.106249998770965526, -2.500000000000000000 ) ) ;
#8763=FACE_OUTER_BOUND ( 'NONE', #5303, .T. ) ;
#8768=CARTESIAN_POINT ( 'NONE',  ( 2.256430356249999658, -3.140624999385482674, -1.302750673588581432 ) ) ;
#8773=CARTESIAN_POINT ( 'NONE',  ( -2.500000000000000000, -1.743749998770965925, 0.000000000000000000 ) ) ;
#8778=CARTESIAN_POINT ( 'NONE',  ( 4.786228327491941173E-16, -3.628124999385482941, 2.605501347177161087 ) ) ;
#8783=CIRCLE ( 'NONE', #1079, 2.500000000000000444 ) ;
#8785=CARTESIAN_POINT ( 'NONE',  ( 2.500000000000000000, -1.931249998770965481, -1.443375672974065438 ) ) ;
#8789=CARTESIAN_POINT ( 'NONE',  ( 5.302876193624534821E-16, -4.387500000000000178, 2.886751345948128655 ) ) ;
#8791=CARTESIAN_POINT ( 'NONE',  ( -2.500000000000000000, -0.3937499987709658922, 0.000000000000000000 ) ) ;
#8792=CARTESIAN_POINT ( 'NONE',  ( -2.256430356249999214, -5.165624999385481253, 1.302750673588581876 ) ) ;
#8793=CYLINDRICAL_SURFACE ( 'NONE', #9272, 2.500000000000000000 ) ;
#8799=CARTESIAN_POINT ( 'NONE',  ( -2.256430356249998770, -4.603124999385482141, 1.302750673588581876 ) ) ;
#8801=ORIENTED_EDGE ( 'NONE', *, *, #6274, .F. ) ;
#8802=CARTESIAN_POINT ( 'NONE',  ( 1.128215178125001161, -3.140624999385482674, 1.954126010382870815 ) ) ;
#8804=( NAMED_UNIT ( * ) PLANE_ANGLE_UNIT ( ) SI_UNIT ( $, .RADIAN. ) );
#8813=VERTEX_POINT ( 'NONE', #6141 ) ;
#8819=CARTESIAN_POINT ( 'NONE',  ( -1.128215178125000273, -3.478124999385482141, -1.954126010382871259 ) ) ;
#8825=CARTESIAN_POINT ( 'NONE',  ( 1.249999999999999334, -1.443749998770965881, -2.165063509461096825 ) ) ;
#8826=ORIENTED_EDGE ( 'NONE', *, *, #3716, .T. ) ;
#8828=DIRECTION ( 'NONE',  ( 0.000000000000000000, -1.000000000000000000, 0.000000000000000000 ) ) ;
#8829=ADVANCED_FACE ( 'NONE', ( #10108 ), #6854, .T. ) ;
#8831=CARTESIAN_POINT ( 'NONE',  ( -1.128215178124998497, -4.115624999385482319, 1.954126010382872147 ) ) ;
#8836=EDGE_CURVE ( 'NONE', #8637, #1444, #575, .T. ) ;
#8839=ORIENTED_EDGE ( 'NONE', *, *, #191, .T. ) ;
#8842=CARTESIAN_POINT ( 'NONE',  ( -3.000000000000000888, -15.00000000000000000, 1.732050807568878303 ) ) ;
#8844=CARTESIAN_POINT ( 'NONE',  ( -2.256430356250000102, -4.753124999385482496, 0.000000000000000000 ) ) ;
#8852=CARTESIAN_POINT ( 'NONE',  ( -2.256430356249998770, -3.253124999385482941, 1.302750673588581876 ) ) ;
#8854=ORIENTED_EDGE ( 'NONE', *, *, #7088, .T. ) ;
#8855=CARTESIAN_POINT ( 'NONE',  ( -2.500000000000000000, -0.03749999999999999167, -1.443375672974064106 ) ) ;
#8863=( BOUNDED_CURVE ( )  B_SPLINE_CURVE ( 2, ( #2710, #404, #5106, #6732, #2764, #8466, #2867, #6050, #9240 ),
 .UNSPECIFIED., .F., .F. ) 
 B_SPLINE_CURVE_WITH_KNOTS ( ( 3, 2, 2, 2, 3 ),
 ( 0.06250000000000000000, 0.06944444444444444753, 0.08333333333333332871, 0.09722222222222222376, 0.1041666666666666713 ),
 .UNSPECIFIED. ) 
 CURVE ( )  GEOMETRIC_REPRESENTATION_ITEM ( )  RATIONAL_B_SPLINE_CURVE ( ( 0.9330127018922194093, 0.9330127018922194093, 1.000000000000000000, 0.8660254037844387076, 1.000000000000000000, 0.8660254037844387076, 1.000000000000000000, 0.9330127018922192983, 0.9330127018922194093 ) ) 
 REPRESENTATION_ITEM ( '' )  );
#8867=PRODUCT_DEFINITION_SHAPE ( 'NONE', 'NONE',  #8713 ) ;
#8869=CARTESIAN_POINT ( 'NONE',  ( 1.128215178125001161, -2.803124999385482319, 1.954126010382870815 ) ) ;
#8872=CARTESIAN_POINT ( 'NONE',  ( 4.996790860652426159E-15, -1.912499999999999867, -2.500000000000000000 ) ) ;
#8873=EDGE_CURVE ( 'NONE', #1383, #3372, #6637, .T. ) ;
#8875=CARTESIAN_POINT ( 'NONE',  ( 2.500000000000000444, -3.806249998770965703, 1.443375672974063439 ) ) ;
#8881=CARTESIAN_POINT ( 'NONE',  ( -2.256430356250000102, -4.228124999385483029, -1.302750673588580321 ) ) ;
#8886=ORIENTED_EDGE ( 'NONE', *, *, #2860, .T. ) ;
#8887=EDGE_CURVE ( 'NONE', #2926, #3621, #6992, .T. ) ;
#8890=CARTESIAN_POINT ( 'NONE',  ( -1.128215178125000273, -0.2156249993854829905, -1.954126010382871259 ) ) ;
#8892=ORIENTED_EDGE ( 'NONE', *, *, #7878, .F. ) ;
#8893=DIRECTION ( 'NONE',  ( 0.000000000000000000, 0.000000000000000000, -1.000000000000000000 ) ) ;
#8900=CARTESIAN_POINT ( 'NONE',  ( 1.128215178124999607, -4.790624999385483029, -1.954126010382871259 ) ) ;
#8903=CARTESIAN_POINT ( 'NONE',  ( -1.128215178124998497, -5.015624999385482674, 1.954126010382872147 ) ) ;
#8904=CYLINDRICAL_SURFACE ( 'NONE', #407, 2.500000000000000000 ) ;
#8907=EDGE_CURVE ( 'NONE', #6136, #3561, #3053, .T. ) ;
#8910=VERTEX_POINT ( 'NONE', #690 ) ;
#8917=CARTESIAN_POINT ( 'NONE',  ( -2.256430356250000102, -3.890624999385481786, -1.302750673588580321 ) ) ;
#8922=( BOUNDED_CURVE ( )  B_SPLINE_CURVE ( 1, ( #8956, #6640 ),
 .UNSPECIFIED., .F., .T. ) 
 B_SPLINE_CURVE_WITH_KNOTS ( ( 2, 2 ),
 ( 0.000000000000000000, 1.000000000000000000 ),
 .UNSPECIFIED. ) 
 CURVE ( )  GEOMETRIC_REPRESENTATION_ITEM ( )  RATIONAL_B_SPLINE_CURVE ( ( 0.9401542295229976531, 0.9401542295229976531 ) ) 
 REPRESENTATION_ITEM ( '' )  );
#8923=CARTESIAN_POINT ( 'NONE',  ( 5.302876193624534821E-16, -4.781249998770966236, 2.886751345948128655 ) ) ;
#8928=CARTESIAN_POINT ( 'NONE',  ( -2.256430356250000102, -4.678124999385483207, -1.302750673588580321 ) ) ;
#8932=CARTESIAN_POINT ( 'NONE',  ( 2.500000000000000444, -3.806249998770965703, 1.443375672974063439 ) ) ;
#8933=ORIENTED_EDGE ( 'NONE', *, *, #4474, .T. ) ;
#8935=FACE_OUTER_BOUND ( 'NONE', #2007, .T. ) ;
#8946=CARTESIAN_POINT ( 'NONE',  ( -1.128215178124998497, -5.015624999385482674, 1.954126010382872147 ) ) ;
#8949=CARTESIAN_POINT ( 'NONE',  ( -2.256430356250000102, -3.778124999385482408, -1.302750673588580321 ) ) ;
#8950=( NAMED_UNIT ( * ) SI_UNIT ( $, .STERADIAN. ) SOLID_ANGLE_UNIT ( ) );
#8956=CARTESIAN_POINT ( 'NONE',  ( -1.728530063377412107, -5.141148402510967053, -1.450400555903694988 ) ) ;
#8963=CARTESIAN_POINT ( 'NONE',  ( 2.500000000000000000, -1.518749998770965837, -3.061616997868383141E-16 ) ) ;
#8967=CARTESIAN_POINT ( 'NONE',  ( 1.128215178125001161, -3.703124999385482230, 1.954126010382870815 ) ) ;
#8972=CARTESIAN_POINT ( 'NONE',  ( -2.256430356250000102, -0.2531249993854829405, 0.000000000000000000 ) ) ;
#8976=DIRECTION ( 'NONE',  ( 0.000000000000000000, -1.000000000000000000, 0.000000000000000000 ) ) ;
#8977=DIRECTION ( 'NONE',  ( 0.08704561088320925122, 0.9949358851208914833, -0.05025580687519624196 ) ) ;
#8993=EDGE_CURVE ( 'NONE', #7561, #9475, #4123, .T. ) ;
#8996=CARTESIAN_POINT ( 'NONE',  ( -3.486133158594716510E-16, -2.362499999999999378, -2.500000000000000000 ) ) ;
#8998=CARTESIAN_POINT ( 'NONE',  ( -1.250000000000000222, -0.07499999999999999722, -2.165063509461096825 ) ) ;
#9000=CARTESIAN_POINT ( 'NONE',  ( -0.6698729810778020211, -2.792403810567666067, -2.500000000000002665 ) ) ;
#9019=CARTESIAN_POINT ( 'NONE',  ( 5.302876193624534821E-16, -3.431249998770965259, 2.886751345948128655 ) ) ;
#9047=CARTESIAN_POINT ( 'NONE',  ( 2.256430356249999658, -4.378124999385482496, -1.302750673588581432 ) ) ;
#9051=EDGE_CURVE ( 'NONE', #4536, #1968, #1172, .T. ) ;
#9054=CARTESIAN_POINT ( 'NONE',  ( -0.6698729810778054627, -0.8075961894323341328, 2.500000000000000000 ) ) ;
#9056=DIRECTION ( 'NONE',  ( 0.000000000000000000, -1.000000000000000000, 0.000000000000000000 ) ) ;
#9062=DIRECTION ( 'NONE',  ( 0.000000000000000000, 0.000000000000000000, -1.000000000000000000 ) ) ;
#9065=CARTESIAN_POINT ( 'NONE',  ( -4.357666448243394824E-15, -2.531249998770965348, 2.500000000000000000 ) ) ;
#9069=( BOUNDED_CURVE ( )  B_SPLINE_CURVE ( 2, ( #7231, #9547, #4728, #4148, #5723, #6454, #167, #6502, #3355 ),
 .UNSPECIFIED., .F., .T. ) 
 B_SPLINE_CURVE_WITH_KNOTS ( ( 3, 2, 2, 2, 3 ),
 ( 0.6041666666666667407, 0.6111111111111111605, 0.6250000000000000000, 0.6388888888888888395, 0.6458333333333333703 ),
 .UNSPECIFIED. ) 
 CURVE ( )  GEOMETRIC_REPRESENTATION_ITEM ( )  RATIONAL_B_SPLINE_CURVE ( ( 0.9330127018922192983, 0.9330127018922198534, 1.000000000000000000, 0.8660254037844387076, 1.000000000000000000, 0.8660254037844387076, 1.000000000000000000, 0.9330127018922187432, 0.9330127018922192983 ) ) 
 REPRESENTATION_ITEM ( '' )  );
#9073=CARTESIAN_POINT ( 'NONE',  ( 1.249999999999999334, -3.693749998770965437, -2.165063509461096825 ) ) ;
#9074=VERTEX_POINT ( 'NONE', #502 ) ;
#9078=LINE ( 'NONE', #5194, #883 ) ;
#9084=FACE_OUTER_BOUND ( 'NONE', #8467, .T. ) ;
#9090=ORIENTED_EDGE ( 'NONE', *, *, #8242, .F. ) ;
#9093=DIRECTION ( 'NONE',  ( 0.000000000000000000, -1.000000000000000000, 0.000000000000000000 ) ) ;
#9097=DIRECTION ( 'NONE',  ( 0.000000000000000000, -1.000000000000000000, 0.000000000000000000 ) ) ;
#9098=CARTESIAN_POINT ( 'NONE',  ( 4.786228327491940187E-16, -4.978124999385483029, 2.605501347177161087 ) ) ;
#9099=CARTESIAN_POINT ( 'NONE',  ( -2.500000000000000000, -2.737499999999999822, -1.443375672974064106 ) ) ;
#9101=CARTESIAN_POINT ( 'NONE',  ( -1.595409442497313560E-16, -0.3656249993854829294, -2.605501347177161087 ) ) ;
#9108=ORIENTED_EDGE ( 'NONE', *, *, #9605, .F. ) ;
#9110=DIRECTION ( 'NONE',  ( 0.04357787137382919396, -0.9961946980917455452, -0.07547908730517349785 ) ) ;
#9114=CARTESIAN_POINT ( 'NONE',  ( 4.786228327491940187E-16, -5.090624999385482852, 2.605501347177161087 ) ) ;
#9119=AXIS2_PLACEMENT_3D ( 'NONE', #6733, #9873, #2521 ) ;
#9121=CARTESIAN_POINT ( 'NONE',  ( -2.256430356249999214, -2.915624999385482585, 1.302750673588581876 ) ) ;
#9125=PLANE ( 'NONE',  #4634 ) ;
#9127=( BOUNDED_CURVE ( )  B_SPLINE_CURVE ( 2, ( #2225, #10066, #1274, #7656, #1994, #6087, #5368, #2053, #3020 ),
 .UNSPECIFIED., .F., .F. ) 
 B_SPLINE_CURVE_WITH_KNOTS ( ( 3, 2, 2, 2, 3 ),
 ( 0.1041666666666666713, 0.1111111111111111049, 0.1250000000000000000, 0.1388888888888888951, 0.1458333333333333426 ),
 .UNSPECIFIED. ) 
 CURVE ( )  GEOMETRIC_REPRESENTATION_ITEM ( )  RATIONAL_B_SPLINE_CURVE ( ( 0.9330127018922194093, 0.9330127018922194093, 1.000000000000000000, 0.8660254037844387076, 1.000000000000000000, 0.8660254037844387076, 1.000000000000000000, 0.9330127018922194093, 0.9330127018922194093 ) ) 
 REPRESENTATION_ITEM ( '' )  );
#9131=CARTESIAN_POINT ( 'NONE',  ( -2.499999999999999556, -0.8062499987709659255, 1.443375672974065882 ) ) ;
#9134=ORIENTED_EDGE ( 'NONE', *, *, #7239, .F. ) ;
#9135=CARTESIAN_POINT ( 'NONE',  ( 0.000000000000000000, 0.000000000000000000, 0.000000000000000000 ) ) ;
#9140=ORIENTED_EDGE ( 'NONE', *, *, #4805, .T. ) ;
#9146=CYLINDRICAL_SURFACE ( 'NONE', #7554, 2.500000000000000000 ) ;
#9147=EDGE_CURVE ( 'NONE', #5722, #7134, #6878, .T. ) ;
#9151=CARTESIAN_POINT ( 'NONE',  ( -9.703070624755296135E-15, -4.837500000000001243, 2.500000000000000444 ) ) ;
#9152=EDGE_LOOP ( 'NONE', ( #9597, #4833, #7003, #308 ) ) ;
#9153=CARTESIAN_POINT ( 'NONE',  ( 2.500000000000000444, -1.162499999999999645, 1.443375672974063439 ) ) ;
#9155=CARTESIAN_POINT ( 'NONE',  ( 2.256430356249999658, -0.4406249993854829961, -1.302750673588581432 ) ) ;
#9158=CARTESIAN_POINT ( 'NONE',  ( -0.6698729810778054627, -1.257596189432333977, 2.500000000000000000 ) ) ;
#9164=CARTESIAN_POINT ( 'NONE',  ( -1.595409442497313560E-16, -0.7031249993854827851, -2.605501347177161087 ) ) ;
#9172=CARTESIAN_POINT ( 'NONE',  ( 2.256430356249999658, -2.690624999385482941, -1.302750673588581432 ) ) ;
#9175=CARTESIAN_POINT ( 'NONE',  ( 9.877377282685029372E-16, -1.631249998770965659, 2.500000000000000000 ) ) ;
#9198=CARTESIAN_POINT ( 'NONE',  ( 5.302876193624534821E-16, -2.137499999999999734, 2.886751345948128655 ) ) ;
#9200=CARTESIAN_POINT ( 'NONE',  ( -2.256430356250000102, -2.540624999385482141, -1.302750673588580321 ) ) ;
#9206=CARTESIAN_POINT ( 'NONE',  ( -2.256430356250000102, -0.1406249993854829794, 0.000000000000000000 ) ) ;
#9207=DIRECTION ( 'NONE',  ( -0.4980973490458728836, -0.08715574274765837404, 0.8627299156628208676 ) ) ;
#9208=CARTESIAN_POINT ( 'NONE',  ( -1.249999999999998224, -1.218749998770965792, 2.165063509461097713 ) ) ;
#9216=VERTEX_POINT ( 'NONE', #3748 ) ;
#9218=CARTESIAN_POINT ( 'NONE',  ( -2.256430356250000102, -2.953124999385482674, 0.000000000000000000 ) ) ;
#9219=EDGE_LOOP ( 'NONE', ( #3078, #34, #4234, #5715 ) ) ;
#9221=CARTESIAN_POINT ( 'NONE',  ( 0.000000000000000000, 0.000000000000000000, -2.500000000000000000 ) ) ;
#9222=CARTESIAN_POINT ( 'NONE',  ( -2.256430356250000102, -0.2531249993854829405, 0.000000000000000000 ) ) ;
#9230=ORIENTED_EDGE ( 'NONE', *, *, #9274, .T. ) ;
#9238=( BOUNDED_CURVE ( )  B_SPLINE_CURVE ( 2, ( #6405, #4052, #9693, #2483, #7234, #5676, #127, #10341, #7287 ),
 .UNSPECIFIED., .F., .F. ) 
 B_SPLINE_CURVE_WITH_KNOTS ( ( 3, 2, 2, 2, 3 ),
 ( 0.8541666666666667407, 0.8611111111111111605, 0.8750000000000000000, 0.8888888888888888395, 0.8958333333333333703 ),
 .UNSPECIFIED. ) 
 CURVE ( )  GEOMETRIC_REPRESENTATION_ITEM ( )  RATIONAL_B_SPLINE_CURVE ( ( 0.9330127018922192983, 0.9330127018922198534, 1.000000000000000000, 0.8660254037844387076, 1.000000000000000000, 0.8660254037844387076, 1.000000000000000000, 0.9330127018922187432, 0.9330127018922192983 ) ) 
 REPRESENTATION_ITEM ( '' )  );
#9240=CARTESIAN_POINT ( 'NONE',  ( 1.045839947578414805E-15, -0.5625000000000001110, -2.500000000000000000 ) ) ;
#9246=CARTESIAN_POINT ( 'NONE',  ( -1.250000000000000222, -2.324999999999999734, -2.165063509461096825 ) ) ;
#9249=CARTESIAN_POINT ( 'NONE',  ( 0.000000000000000000, -20.00000000000000000, 0.000000000000000000 ) ) ;
#9250=CARTESIAN_POINT ( 'NONE',  ( -1.595409442497313560E-16, -0.8156249993854829405, -2.605501347177161087 ) ) ;
#9254=VERTEX_POINT ( 'NONE', #4744 ) ;
#9261=CARTESIAN_POINT ( 'NONE',  ( -1.128215178125000273, -0.6656249993854830294, -1.954126010382871259 ) ) ;
#9264=CARTESIAN_POINT ( 'NONE',  ( -2.378215178125000495, -0.07031249969274147582, 0.000000000000000000 ) ) ;
#9272=AXIS2_PLACEMENT_3D ( 'NONE', #736, #4132, #8893 ) ;
#9274=EDGE_CURVE ( 'NONE', #1968, #4141, #1895, .T. ) ;
#9275=CARTESIAN_POINT ( 'NONE',  ( 1.128215178124999607, -2.653124999385482408, -1.954126010382871259 ) ) ;
#9281=CARTESIAN_POINT ( 'NONE',  ( -1.128215178125000273, -0.7781249993854828517, -1.954126010382871259 ) ) ;
#9291=CARTESIAN_POINT ( 'NONE',  ( -2.256430356249999214, -1.903124999385482852, 1.302750673588581876 ) ) ;
#9294=CARTESIAN_POINT ( 'NONE',  ( -2.500000000000000000, -0.8437499987709659033, 0.000000000000000000 ) ) ;
#9296=CARTESIAN_POINT ( 'NONE',  ( 0.000000000000000000, 0.000000000000000000, -0.4999999999999953371 ) ) ;
#9297=DIRECTION ( 'NONE',  ( 0.000000000000000000, -1.000000000000000000, 0.000000000000000000 ) ) ;
#9298=ORIENTED_EDGE ( 'NONE', *, *, #3321, .T. ) ;
#9304=CARTESIAN_POINT ( 'NONE',  ( -1.250000000000000222, -0.5250000000000000222, -2.165063509461096825 ) ) ;
#9308=CARTESIAN_POINT ( 'NONE',  ( -2.256430356250000102, -2.953124999385482674, 0.000000000000000000 ) ) ;
#9320=CARTESIAN_POINT ( 'NONE',  ( -1.595409442497313560E-16, -1.603124999385482807, -2.605501347177161087 ) ) ;
#9321=CARTESIAN_POINT ( 'NONE',  ( -2.499999999999999112, -5.306249998770965703, 1.443375672974065882 ) ) ;
#9323=FACE_OUTER_BOUND ( 'NONE', #400, .T. ) ;
#9331=ORIENTED_EDGE ( 'NONE', *, *, #9777, .T. ) ;
#9336=CARTESIAN_POINT ( 'NONE',  ( -1.128215178124998497, -1.528124999385482852, 1.954126010382872147 ) ) ;
#9343=CARTESIAN_POINT ( 'NONE',  ( 1.128215178124999607, -2.203124999385482674, -1.954126010382871259 ) ) ;
#9347=DIRECTION ( 'NONE',  ( 0.000000000000000000, -1.000000000000000000, 0.000000000000000000 ) ) ;
#9349=CARTESIAN_POINT ( 'NONE',  ( 9.877377282685029372E-16, -3.037499999999999201, 2.500000000000000000 ) ) ;
#9350=VERTEX_POINT ( 'NONE', #8095 ) ;
#9351=CARTESIAN_POINT ( 'NONE',  ( 0.6698729810778075722, -1.217403810567665667, 2.499999999999999556 ) ) ;
#9352=CARTESIAN_POINT ( 'NONE',  ( 1.034219503716432668E-14, -4.162500000000000533, -2.500000000000000000 ) ) ;
#9353=CARTESIAN_POINT ( 'NONE',  ( -1.128215178124998497, -0.5156249993854828961, 1.954126010382872147 ) ) ;
#9357=EDGE_CURVE ( 'NONE', #1260, #4596, #5637, .T. ) ;
#9363=CARTESIAN_POINT ( 'NONE',  ( -4.357666448243394824E-15, -2.981249998770965526, 2.500000000000000000 ) ) ;
#9366=CARTESIAN_POINT ( 'NONE',  ( 5.302876193624534821E-16, -3.487499999999999822, 2.886751345948128655 ) ) ;
#9368=CARTESIAN_POINT ( 'NONE',  ( -1.868473738487927527, -5.035679442772306835, -1.567817502008199249 ) ) ;
#9369=CARTESIAN_POINT ( 'NONE',  ( 2.256430356249999658, -2.240624999385482319, -1.302750673588581432 ) ) ;
#9376=CARTESIAN_POINT ( 'NONE',  ( 0.000000000000000000, 0.000000000000000000, 0.000000000000000000 ) ) ;
#9378=CARTESIAN_POINT ( 'NONE',  ( 2.256430356249999658, -1.228124999385483029, -1.302750673588581432 ) ) ;
#9380=ORIENTED_EDGE ( 'NONE', *, *, #2624, .F. ) ;
#9387=ORIENTED_EDGE ( 'NONE', *, *, #7878, .T. ) ;
#9391=CARTESIAN_POINT ( 'NONE',  ( -1.128215178125000273, -3.028124999385482408, -1.954126010382871259 ) ) ;
#9398=CARTESIAN_POINT ( 'NONE',  ( -1.128215178125000273, -2.128124999385482496, -1.954126010382871259 ) ) ;
#9403=CARTESIAN_POINT ( 'NONE',  ( -2.500000000000000000, -3.131249998770965437, -1.443375672974064106 ) ) ;
#9408=CARTESIAN_POINT ( 'NONE',  ( 1.128215178124999607, -2.540624999385482585, -1.954126010382871259 ) ) ;
#9416=EDGE_CURVE ( 'NONE', #7920, #4798, #3441, .T. ) ;
#9422=ADVANCED_FACE ( 'NONE', ( #1657, #384 ), #9125, .F. ) ;
#9423=CARTESIAN_POINT ( 'NONE',  ( -1.249999999999998224, -3.074999999999999734, 2.165063509461097713 ) ) ;
#9426=CARTESIAN_POINT ( 'NONE',  ( 1.128215178125001161, -1.003124999385482718, 1.954126010382870815 ) ) ;
#9430=EDGE_LOOP ( 'NONE', ( #9090, #193, #7056, #6030 ) ) ;
#9435=CARTESIAN_POINT ( 'NONE',  ( -1.128215178125000273, -1.565624999385482941, -1.954126010382871259 ) ) ;
#9439=CARTESIAN_POINT ( 'NONE',  ( 2.256430356250000546, -1.753124999385482718, 1.302750673588579877 ) ) ;
#9449=CARTESIAN_POINT ( 'NONE',  ( 2.256430356250000546, -3.665624999385482141, 1.302750673588579877 ) ) ;
#9450=ORIENTED_EDGE ( 'NONE', *, *, #2670, .F. ) ;
#9456=CARTESIAN_POINT ( 'NONE',  ( -2.256430356249998770, -0.6656249993854829183, 1.302750673588581876 ) ) ;
#9460=CARTESIAN_POINT ( 'NONE',  ( -2.499999999999999556, -1.706249998770965615, 1.443375672974065882 ) ) ;
#9461=ORIENTED_EDGE ( 'NONE', *, *, #914, .T. ) ;
#9465=CARTESIAN_POINT ( 'NONE',  ( 2.256430356250000546, -0.8531249993854829183, 1.302750673588579877 ) ) ;
#9466=ORIENTED_EDGE ( 'NONE', *, *, #3951, .F. ) ;
#9471=CARTESIAN_POINT ( 'NONE',  ( -2.793760218496626182E-16, -25.00000000000000000, 2.062556682370379590 ) ) ;
#9475=VERTEX_POINT ( 'NONE', #2740 ) ;
#9476=CARTESIAN_POINT ( 'NONE',  ( 1.249999999999999334, -3.299999999999999378, -2.165063509461096825 ) ) ;
#9479=CARTESIAN_POINT ( 'NONE',  ( 1.128215178125001161, -3.703124999385482230, 1.954126010382870815 ) ) ;
#9490=CARTESIAN_POINT ( 'NONE',  ( -2.256430356250000102, -4.678124999385483207, -1.302750673588580321 ) ) ;
#9492=CARTESIAN_POINT ( 'NONE',  ( -1.595409442497313560E-16, -2.503124999385482496, -2.605501347177161087 ) ) ;
#9496=CARTESIAN_POINT ( 'NONE',  ( 0.6698729810778063509, -2.776346188203299814, -2.500000000000000000 ) ) ;
#9500=ORIENTED_EDGE ( 'NONE', *, *, #7604, .T. ) ;
#9503=CARTESIAN_POINT ( 'NONE',  ( 2.256430356250000102, -3.628124999385482496, -2.763330213280484622E-16 ) ) ;
#9508=CARTESIAN_POINT ( 'NONE',  ( -1.128215178124998497, -1.528124999385482852, 1.954126010382872147 ) ) ;
#9510=CARTESIAN_POINT ( 'NONE',  ( -2.256430356250000102, -0.2531249993854829405, 0.000000000000000000 ) ) ;
#9512=CARTESIAN_POINT ( 'NONE',  ( 2.500000000000000000, -2.831249998770965615, -1.443375672974064994 ) ) ;
#9516=CARTESIAN_POINT ( 'NONE',  ( 1.128215178125001161, -1.790624999385482807, 1.954126010382870815 ) ) ;
#9519=ORIENTED_EDGE ( 'NONE', *, *, #6569, .F. ) ;
#9520=CARTESIAN_POINT ( 'NONE',  ( 9.877377282685029372E-16, -1.237499999999999600, 2.500000000000000000 ) ) ;
#9522=CARTESIAN_POINT ( 'NONE',  ( -1.250000000000000222, -3.618749998770965259, -2.165063509461096825 ) ) ;
#9526=CARTESIAN_POINT ( 'NONE',  ( 2.500000000000000444, -4.312499999999999112, 1.443375672974063439 ) ) ;
#9528=EDGE_CURVE ( 'NONE', #7541, #3111, #9707, .T. ) ;
#9530=CARTESIAN_POINT ( 'NONE',  ( -2.256430356249999214, -4.265624999385482674, 1.302750673588581876 ) ) ;
#9538=CARTESIAN_POINT ( 'NONE',  ( -2.256430356250000102, -4.190624999385482496, 0.000000000000000000 ) ) ;
#9541=CARTESIAN_POINT ( 'NONE',  ( -2.256430356249999214, -3.253124999385482941, 1.302750673588581876 ) ) ;
#9547=CARTESIAN_POINT ( 'NONE',  ( 0.6698729810778112359, -3.282596189432334111, -2.499999999999996447 ) ) ;
#9550=CARTESIAN_POINT ( 'NONE',  ( 1.128215178124999607, -4.903124999385481964, -1.954126010382871259 ) ) ;
#9551=ORIENTED_EDGE ( 'NONE', *, *, #9811, .F. ) ;
#9556=CARTESIAN_POINT ( 'NONE',  ( -1.595409442497313560E-16, -3.515624999385482674, -2.605501347177161087 ) ) ;
#9560=CARTESIAN_POINT ( 'NONE',  ( 2.500000000000000000, -3.318749998770965437, -3.061616997868383141E-16 ) ) ;
#9561=VERTEX_POINT ( 'NONE', #9175 ) ;
#9565=CARTESIAN_POINT ( 'NONE',  ( 2.256430356250000546, -3.103124999385482585, 1.302750673588579877 ) ) ;
#9566=ORIENTED_EDGE ( 'NONE', *, *, #121, .T. ) ;
#9572=CARTESIAN_POINT ( 'NONE',  ( -2.499999999999999556, -3.562500000000000444, 1.443375672974065882 ) ) ;
#9574=CARTESIAN_POINT ( 'NONE',  ( -2.256430356249999214, -4.715624999385481964, 1.302750673588581876 ) ) ;
#9583=CARTESIAN_POINT ( 'NONE',  ( 2.256430356250000102, -3.065624999385482496, -2.763330213280484622E-16 ) ) ;
#9584=CARTESIAN_POINT ( 'NONE',  ( 0.000000000000000000, -25.00000000000000000, -0.4999999999999953371 ) ) ;
#9585=CARTESIAN_POINT ( 'NONE',  ( 1.128215178125001161, -1.340624999385482852, 1.954126010382870815 ) ) ;
#9595=( BOUNDED_CURVE ( )  B_SPLINE_CURVE ( 2, ( #1967, #1192, #5850, #7322, #6538 ),
 .UNSPECIFIED., .F., .F. ) 
 B_SPLINE_CURVE_WITH_KNOTS ( ( 3, 2, 3 ),
 ( 0.000000000000000000, 0.01388888888888888985, 0.02083333333333333565 ),
 .UNSPECIFIED. ) 
 CURVE ( )  GEOMETRIC_REPRESENTATION_ITEM ( )  RATIONAL_B_SPLINE_CURVE ( ( 1.000000000000000000, 0.8660254037844387076, 1.000000000000000000, 0.9330127018922192983, 0.9330127018922194093 ) ) 
 REPRESENTATION_ITEM ( '' )  );
#9596=CARTESIAN_POINT ( 'NONE',  ( 4.786228327491941173E-16, -4.640624999385482674, 2.605501347177161087 ) ) ;
#9597=ORIENTED_EDGE ( 'NONE', *, *, #5985, .F. ) ;
#9601=CARTESIAN_POINT ( 'NONE',  ( 1.128215178124999607, -4.903124999385481964, -1.954126010382871259 ) ) ;
#9605=EDGE_CURVE ( 'NONE', #6035, #4027, #9127, .T. ) ;
#9606=EDGE_CURVE ( 'NONE', #9074, #7561, #2847, .T. ) ;
#9607=CARTESIAN_POINT ( 'NONE',  ( -1.250000000000000222, -1.368749998770965925, -2.165063509461096825 ) ) ;
#9612=CARTESIAN_POINT ( 'NONE',  ( -2.256430356249999658, -5.114265559567681585, -0.8212734853698877568 ) ) ;
#9626=CARTESIAN_POINT ( 'NONE',  ( 2.256430356250000102, -4.528124999385481964, -2.763330213280484622E-16 ) ) ;
#9629=CARTESIAN_POINT ( 'NONE',  ( -4.357666448243394824E-15, -2.137500000000000178, 2.500000000000000000 ) ) ;
#9633=CARTESIAN_POINT ( 'NONE',  ( 2.256430356249999658, -3.028124999385482852, -1.302750673588581432 ) ) ;
#9636=CARTESIAN_POINT ( 'NONE',  ( -1.595409442497313560E-16, -2.053124999385482763, -2.605501347177161087 ) ) ;
#9640=EDGE_CURVE ( 'NONE', #2167, #3761, #7598, .T. ) ;
#9650=CARTESIAN_POINT ( 'NONE',  ( -1.128215178124998497, -3.328124999385482230, 1.954126010382872147 ) ) ;
#9656=( BOUNDED_CURVE ( )  B_SPLINE_CURVE ( 2, ( #2212, #9496, #10114, #5415, #2951, #6242, #2157, #5359, #7815 ),
 .UNSPECIFIED., .F., .T. ) 
 B_SPLINE_CURVE_WITH_KNOTS ( ( 3, 2, 2, 2, 3 ),
 ( 0.4375000000000000000, 0.4444444444444444198, 0.4583333333333333148, 0.4722222222222222099, 0.4791666666666666852 ),
 .UNSPECIFIED. ) 
 CURVE ( )  GEOMETRIC_REPRESENTATION_ITEM ( )  RATIONAL_B_SPLINE_CURVE ( ( 0.9330127018922194093, 0.9330127018922194093, 1.000000000000000000, 0.8660254037844387076, 1.000000000000000000, 0.8660254037844387076, 1.000000000000000000, 0.9330127018922190762, 0.9330127018922194093 ) ) 
 REPRESENTATION_ITEM ( '' )  );
#9658=CARTESIAN_POINT ( 'NONE',  ( 5.302876193624534821E-16, -3.881249998770965437, 2.886751345948128655 ) ) ;
#9663=CARTESIAN_POINT ( 'NONE',  ( -1.595409442497313560E-16, -4.753124999385481608, -2.605501347177161087 ) ) ;
#9668=CARTESIAN_POINT ( 'NONE',  ( 9.877377282685029372E-16, -2.081249998770965615, 2.500000000000000000 ) ) ;
#9674=CARTESIAN_POINT ( 'NONE',  ( -2.256430356250000102, -3.853124999385482585, 0.000000000000000000 ) ) ;
#9682=CARTESIAN_POINT ( 'NONE',  ( -1.128215178125000273, -4.715624999385481964, -1.954126010382871259 ) ) ;
#9683=CARTESIAN_POINT ( 'NONE',  ( 2.500000000000000000, -2.437500000000000000, -1.443375672974065438 ) ) ;
#9685=CARTESIAN_POINT ( 'NONE',  ( -1.128215178125000273, -3.815624999385482941, -1.954126010382871259 ) ) ;
#9693=CARTESIAN_POINT ( 'NONE',  ( 1.249999999999999334, -5.043749998770965526, -2.165063509461096825 ) ) ;
#9697=CARTESIAN_POINT ( 'NONE',  ( 2.256430356250000102, -4.078124999385482674, -2.763330213280484622E-16 ) ) ;
#9702=CARTESIAN_POINT ( 'NONE',  ( 2.500000000000000000, -5.081249998770965171, -1.443375672974064994 ) ) ;
#9707=LINE ( 'NONE', #2545, #7300 ) ;
#9709=CARTESIAN_POINT ( 'NONE',  ( -1.128215178125000273, -4.265624999385482674, -1.954126010382871259 ) ) ;
#9713=FACE_OUTER_BOUND ( 'NONE', #6981, .T. ) ;
#9722=CARTESIAN_POINT ( 'NONE',  ( 0.6698729810778075722, -4.761153809338632747, 2.499999999999999556 ) ) ;
#9728=VERTEX_POINT ( 'NONE', #5914 ) ;
#9729=CARTESIAN_POINT ( 'NONE',  ( 2.256430356250000102, -4.865624999385482319, -2.763330213280484622E-16 ) ) ;
#9730=( NAMED_UNIT ( * ) PLANE_ANGLE_UNIT ( ) SI_UNIT ( $, .RADIAN. ) );
#9732=CARTESIAN_POINT ( 'NONE',  ( -2.256430356249999214, -0.6656249993854828073, 1.302750673588581876 ) ) ;
#9736=SHAPE_REPRESENTATION ( 'grease nipple', ( #5055 ), #7312 ) ;
#9740=STYLED_ITEM('',(#10394),#2806);
#9742=VECTOR ( 'NONE', #4527, 1000.000000000000000 ) ;
#9744=DIRECTION ( 'NONE',  ( 1.000000000000000000, 0.000000000000000000, 0.000000000000000000 ) ) ;
#9745=CARTESIAN_POINT ( 'NONE',  ( -1.128215178124998497, -2.878124999385482496, 1.954126010382872147 ) ) ;
#9750=CARTESIAN_POINT ( 'NONE',  ( -1.767625397874844694E-16, -4.106249998770965526, -2.886751345948128655 ) ) ;
#9756=CARTESIAN_POINT ( 'NONE',  ( -2.256430356250000102, -3.290624999385482585, 0.000000000000000000 ) ) ;
#9762=CARTESIAN_POINT ( 'NONE',  ( -2.500000000000000000, -4.500000000000000000, 0.000000000000000000 ) ) ;
#9765=EDGE_CURVE ( 'NONE', #10197, #4536, #3359, .T. ) ;
#9769=PLANE ( 'NONE',  #7695 ) ;
#9771=DIRECTION ( 'NONE',  ( 0.000000000000000000, 0.000000000000000000, -1.000000000000000000 ) ) ;
#9773=CARTESIAN_POINT ( 'NONE',  ( 0.6698729810778025762, -4.817403810567666866, 2.500000000000002665 ) ) ;
#9776=CARTESIAN_POINT ( 'NONE',  ( -0.7001057366827120321, -5.193520385083734148, -2.676043109347841398 ) ) ;
#9777=EDGE_CURVE ( 'NONE', #5851, #9561, #859, .T. ) ;
#9794=VECTOR ( 'NONE', #4632, 1000.000000000000000 ) ;
#9798=CARTESIAN_POINT ( 'NONE',  ( -1.767625397874844694E-16, -5.006249998770964993, -2.886751345948128655 ) ) ;
#9802=DIRECTION ( 'NONE',  ( 0.000000000000000000, 0.000000000000000000, -1.000000000000000000 ) ) ;
#9809=CARTESIAN_POINT ( 'NONE',  ( -3.000000000000000888, -15.00000000000000000, 1.732050807568878303 ) ) ;
#9810=ORIENTED_EDGE ( 'NONE', *, *, #9640, .F. ) ;
#9811=EDGE_CURVE ( 'NONE', #2830, #5851, #10145, .T. ) ;
#9814=CARTESIAN_POINT ( 'NONE',  ( -1.249999999999998224, -2.118749998770965703, 2.165063509461097713 ) ) ;
#9822=DIRECTION ( 'NONE',  ( -1.067350013832299517E-17, 0.9961946980917455452, 0.08715574274765836016 ) ) ;
#9824=AXIS2_PLACEMENT_3D ( 'NONE', #809, #9097, #5007 ) ;
#9826=CARTESIAN_POINT ( 'NONE',  ( -2.256430356249999658, -5.114265559567680697, -0.8212734853698876458 ) ) ;
#9830=CARTESIAN_POINT ( 'NONE',  ( 2.500000000000000444, -0.2624999999999999556, 1.443375672974063439 ) ) ;
#9834=CARTESIAN_POINT ( 'NONE',  ( 2.500000000000000000, -0.5812499987709658367, -1.443375672974065438 ) ) ;
#9842=CARTESIAN_POINT ( 'NONE',  ( 0.000000000000000000, 0.000000000000000000, 0.000000000000000000 ) ) ;
#9848=CARTESIAN_POINT ( 'NONE',  ( -2.500000000000000000, -3.581249998770965615, -1.443375672974064106 ) ) ;
#9850=ORIENTED_EDGE ( 'NONE', *, *, #9147, .T. ) ;
#9852=CARTESIAN_POINT ( 'NONE',  ( 0.000000000000000000, 0.000000000000000000, 0.000000000000000000 ) ) ;
#9855=( BOUNDED_CURVE ( )  B_SPLINE_CURVE ( 2, ( #1912, #7318, #5105, #8304, #3343, #4958, #6535, #9722, #987 ),
 .UNSPECIFIED., .F., .F. ) 
 B_SPLINE_CURVE_WITH_KNOTS ( ( 3, 2, 2, 2, 3 ),
 ( 0.7708333333333333703, 0.7777777777777777901, 0.7916666666666666297, 0.8055555555555555802, 0.8125000000000000000 ),
 .UNSPECIFIED. ) 
 CURVE ( )  GEOMETRIC_REPRESENTATION_ITEM ( )  RATIONAL_B_SPLINE_CURVE ( ( 0.9330127018922192983, 0.9330127018922198534, 1.000000000000000000, 0.8660254037844387076, 1.000000000000000000, 0.8660254037844387076, 1.000000000000000000, 0.9330127018922194093, 0.9330127018922194093 ) ) 
 REPRESENTATION_ITEM ( '' )  );
#9873=DIRECTION ( 'NONE',  ( 0.000000000000000000, -1.000000000000000000, 0.000000000000000000 ) ) ;
#9876=CARTESIAN_POINT ( 'NONE',  ( -1.767625397874844694E-16, -2.812500000000000000, -2.886751345948128655 ) ) ;
#9878=CARTESIAN_POINT ( 'NONE',  ( 2.562556682370379146, -20.00000000000000000, -1.732050807568876749 ) ) ;
#9881=AXIS2_PLACEMENT_3D ( 'NONE', #3460, #8275, #9062 ) ;
#9883=ADVANCED_FACE ( 'NONE', ( #1984 ), #3730, .T. ) ;
#9900=FACE_OUTER_BOUND ( 'NONE', #5598, .T. ) ;
#9902=CARTESIAN_POINT ( 'NONE',  ( -1.128215178125000273, -2.128124999385482496, -1.954126010382871259 ) ) ;
#9908=ADVANCED_FACE ( 'NONE', ( #9323 ), #1367, .F. ) ;
#9910=ADVANCED_FACE ( 'NONE', ( #6969 ), #6265, .T. ) ;
#9924=FACE_BOUND ( 'NONE', #3570, .T. ) ;
#9926=CARTESIAN_POINT ( 'NONE',  ( -2.500000000000000000, -4.031249998770966236, -1.443375672974064106 ) ) ;
#9930=ORIENTED_EDGE ( 'NONE', *, *, #5652, .F. ) ;
#9932=CARTESIAN_POINT ( 'NONE',  ( 0.000000000000000000, -15.00000000000000000, 0.000000000000000000 ) ) ;
#9933=CARTESIAN_POINT ( 'NONE',  ( -1.249999999999998224, -2.174999999999999822, 2.165063509461097713 ) ) ;
#9935=CARTESIAN_POINT ( 'NONE',  ( 1.250000000000001110, -2.100000000000000089, 2.165063509461096380 ) ) ;
#9940=CARTESIAN_POINT ( 'NONE',  ( 9.877377282685029372E-16, -0.7874999999999998668, 2.500000000000000000 ) ) ;
#9945=CIRCLE ( 'NONE', #5612, 0.4999999999999953371 ) ;
#9948=EDGE_CURVE ( 'NONE', #8813, #3761, #8641, .T. ) ;
#9949=CARTESIAN_POINT ( 'NONE',  ( -1.250000000000000222, -1.368749998770965925, -2.165063509461096825 ) ) ;
#9957=CARTESIAN_POINT ( 'NONE',  ( 1.128215178125001161, -1.903124999385482852, 1.954126010382870815 ) ) ;
#9958=ORIENTED_EDGE ( 'NONE', *, *, #1522, .F. ) ;
#9961=ADVANCED_FACE ( 'NONE', ( #8935 ), #4997, .T. ) ;
#9976=CARTESIAN_POINT ( 'NONE',  ( -9.703070624755296135E-15, -3.487499999999999822, 2.500000000000000444 ) ) ;
#9981=( BOUNDED_CURVE ( )  B_SPLINE_CURVE ( 2, ( #5966, #9158, #1978, #3354, #4970, #8170, #1824, #5019, #8216 ),
 .UNSPECIFIED., .F., .T. ) 
 B_SPLINE_CURVE_WITH_KNOTS ( ( 3, 2, 2, 2, 3 ),
 ( 0.2291666666666666574, 0.2361111111111111049, 0.2500000000000000000, 0.2638888888888888951, 0.2708333333333333703 ),
 .UNSPECIFIED. ) 
 CURVE ( )  GEOMETRIC_REPRESENTATION_ITEM ( )  RATIONAL_B_SPLINE_CURVE ( ( 0.9330127018922194093, 0.9330127018922194093, 1.000000000000000000, 0.8660254037844387076, 1.000000000000000000, 0.8660254037844387076, 1.000000000000000000, 0.9330127018922190762, 0.9330127018922194093 ) ) 
 REPRESENTATION_ITEM ( '' )  );
#9982=CARTESIAN_POINT ( 'NONE',  ( 0.000000000000000000, 0.000000000000000000, 0.000000000000000000 ) ) ;
#9989=CARTESIAN_POINT ( 'NONE',  ( 1.249999999999999334, -1.949999999999999956, -2.165063509461096825 ) ) ;
#9990=CARTESIAN_POINT ( 'NONE',  ( -1.915121305771201099, 0.000000000000000000, -1.606956870666170323 ) ) ;
#9991=CARTESIAN_POINT ( 'NONE',  ( 4.786228327491941173E-16, -1.940624999385482718, 2.605501347177161087 ) ) ;
#10002=CARTESIAN_POINT ( 'NONE',  ( -2.256430356250000102, -0.6281249993854828295, -1.302750673588580321 ) ) ;
#10009=CARTESIAN_POINT ( 'NONE',  ( -1.595409442497313560E-16, -2.615624999385482319, -2.605501347177161087 ) ) ;
#10018=CARTESIAN_POINT ( 'NONE',  ( -2.499999999999999112, -2.606249998770965526, 1.443375672974065882 ) ) ;
#10020=ORIENTED_EDGE ( 'NONE', *, *, #4409, .T. ) ;
#10023=CARTESIAN_POINT ( 'NONE',  ( -2.500000000000000000, -4.973640350848739899, -0.9099175284171375777 ) ) ;
#10031=EDGE_LOOP ( 'NONE', ( #6760, #4167, #8565, #2549 ) ) ;
#10034=ORIENTED_EDGE ( 'NONE', *, *, #9528, .F. ) ;
#10036=CARTESIAN_POINT ( 'NONE',  ( 1.249999999999999334, -1.050000000000000044, -2.165063509461096825 ) ) ;
#10039=CARTESIAN_POINT ( 'NONE',  ( 2.256430356249999658, -0.8906249993854827851, -1.302750673588581432 ) ) ;
#10043=ADVANCED_FACE ( 'NONE', ( #9084 ), #1902, .T. ) ;
#10045=CARTESIAN_POINT ( 'NONE',  ( -0.6698729810778081273, -3.001346188203299903, 2.499999999999999112 ) ) ;
#10048=VERTEX_POINT ( 'NONE', #2856 ) ;
#10049=CARTESIAN_POINT ( 'NONE',  ( 2.256430356250000102, -2.165624999385483029, -2.763330213280484622E-16 ) ) ;
#10056=VECTOR ( 'NONE', #7546, 1000.000000000000114 ) ;
#10060=ORIENTED_EDGE ( 'NONE', *, *, #6418, .F. ) ;
#10062=CARTESIAN_POINT ( 'NONE',  ( -1.728530063377412107, -5.141148402510967053, -1.450400555903694988 ) ) ;
#10063=CARTESIAN_POINT ( 'NONE',  ( -2.256430356249999214, -1.565624999385482718, 1.302750673588581876 ) ) ;
#10066=CARTESIAN_POINT ( 'NONE',  ( 0.6698729810778069060, -0.5825961894323341550, -2.500000000000000000 ) ) ;
#10068=CARTESIAN_POINT ( 'NONE',  ( -1.128215178125000273, -0.3281249993854828961, -1.954126010382871259 ) ) ;
#10069=CARTESIAN_POINT ( 'NONE',  ( -2.562556682370380035, -20.00000000000000000, 1.732050807568878303 ) ) ;
#10070=VECTOR ( 'NONE', #8503, 1000.000000000000000 ) ;
#10072=CARTESIAN_POINT ( 'NONE',  ( 0.000000000000000000, 0.000000000000000000, 0.000000000000000000 ) ) ;
#10073=CARTESIAN_POINT ( 'NONE',  ( -1.250000000000000222, -2.718749998770965792, -2.165063509461096825 ) ) ;
#10075=ORIENTED_EDGE ( 'NONE', *, *, #9606, .T. ) ;
#10079=CARTESIAN_POINT ( 'NONE',  ( 4.786228327491941173E-16, -0.9281249993854828739, 2.605501347177161087 ) ) ;
#10081=LINE ( 'NONE', #6827, #4259 ) ;
#10084=PLANE ( 'NONE',  #7373 ) ;
#10085=LINE ( 'NONE', #2921, #6367 ) ;
#10086=CARTESIAN_POINT ( 'NONE',  ( 0.000000000000000000, 0.000000000000000000, 0.000000000000000000 ) ) ;
#10091=CARTESIAN_POINT ( 'NONE',  ( -2.500000000000000000, -1.387499999999999956, -1.443375672974064106 ) ) ;
#10093=DIRECTION ( 'NONE',  ( -0.000000000000000000, 1.000000000000000000, -0.000000000000000000 ) ) ;
#10094=CARTESIAN_POINT ( 'NONE',  ( -1.128215178124998497, -1.978124999385482807, 1.954126010382872147 ) ) ;
#10099=CARTESIAN_POINT ( 'NONE',  ( 2.500000000000000444, -2.062499999999999556, 1.443375672974063439 ) ) ;
#10105=DIRECTION ( 'NONE',  ( 0.000000000000000000, 0.000000000000000000, -1.000000000000000000 ) ) ;
#10106=EDGE_LOOP ( 'NONE', ( #8801, #654, #6778, #2036 ) ) ;
#10107=CARTESIAN_POINT ( 'NONE',  ( -2.256430356250000102, -1.978124999385482807, -1.302750673588580321 ) ) ;
#10108=FACE_OUTER_BOUND ( 'NONE', #7699, .T. ) ;
#10111=DIRECTION ( 'NONE',  ( -0.04357787137382917314, -0.9961946980917455452, -0.07547908730517351172 ) ) ;
#10114=CARTESIAN_POINT ( 'NONE',  ( 1.249999999999999334, -2.793749998770965526, -2.165063509461096825 ) ) ;
#10117=ORIENTED_EDGE ( 'NONE', *, *, #9606, .F. ) ;
#10118=VECTOR ( 'NONE', #5565, 1000.000000000000000 ) ;
#10121=CARTESIAN_POINT ( 'NONE',  ( 1.128215178124999607, -0.8531249993854828073, -1.954126010382871259 ) ) ;
#10128=CARTESIAN_POINT ( 'NONE',  ( 2.256430356250000546, -1.865624999385482985, 1.302750673588579877 ) ) ;
#10129=LINE ( 'NONE', #10069, #4372 ) ;
#10134=CARTESIAN_POINT ( 'NONE',  ( -4.357666448243394824E-15, -2.531249998770965348, 2.500000000000000000 ) ) ;
#10138=CARTESIAN_POINT ( 'NONE',  ( 1.249999999999999334, -4.200000000000000178, -2.165063509461096825 ) ) ;
#10139=CARTESIAN_POINT ( 'NONE',  ( -1.128215178125000273, -2.465624999385482852, -1.954126010382871259 ) ) ;
#10142=CYLINDRICAL_SURFACE ( 'NONE', #5253, 0.4999999999999953371 ) ;
#10143=VECTOR ( 'NONE', #8130, 1000.000000000000000 ) ;
#10145=( BOUNDED_CURVE ( )  B_SPLINE_CURVE ( 2, ( #1157, #6912, #9208, #1208, #6073, #1317, #9949, #7758, #4402 ),
 .UNSPECIFIED., .F., .T. ) 
 B_SPLINE_CURVE_WITH_KNOTS ( ( 3, 2, 2, 2, 3 ),
 ( 0.1458333333333333426, 0.1527777777777777901, 0.1666666666666666574, 0.1805555555555555525, 0.1875000000000000000 ),
 .UNSPECIFIED. ) 
 CURVE ( )  GEOMETRIC_REPRESENTATION_ITEM ( )  RATIONAL_B_SPLINE_CURVE ( ( 0.9330127018922194093, 0.9330127018922194093, 1.000000000000000000, 0.8660254037844387076, 1.000000000000000000, 0.8660254037844387076, 1.000000000000000000, 0.9330127018922194093, 0.9330127018922194093 ) ) 
 REPRESENTATION_ITEM ( '' )  );
#10151=ORIENTED_EDGE ( 'NONE', *, *, #6453, .T. ) ;
#10155=CARTESIAN_POINT ( 'NONE',  ( 2.500000000000000000, -2.924999999999999822, -3.061616997868383141E-16 ) ) ;
#10158=CARTESIAN_POINT ( 'NONE',  ( 1.128215178124999607, -1.303124999385482985, -1.954126010382871259 ) ) ;
#10162=CARTESIAN_POINT ( 'NONE',  ( -1.249999999999998224, -3.524999999999999467, 2.165063509461097713 ) ) ;
#10167=CARTESIAN_POINT ( 'NONE',  ( 2.256430356250000102, -1.265624999385482896, -2.763330213280484622E-16 ) ) ;
#10168=DIRECTION ( 'NONE',  ( -0.000000000000000000, -1.000000000000000000, -0.000000000000000000 ) ) ;
#10170=CARTESIAN_POINT ( 'NONE',  ( -1.128215178125000273, -0.2156249993854829350, -1.954126010382871259 ) ) ;
#10177=VERTEX_POINT ( 'NONE', #1285 ) ;
#10179=CARTESIAN_POINT ( 'NONE',  ( 0.000000000000000000, -15.00000000000000000, 0.000000000000000000 ) ) ;
#10180=ORIENTED_EDGE ( 'NONE', *, *, #4726, .T. ) ;
#10181=CARTESIAN_POINT ( 'NONE',  ( -2.256430356249999214, -3.815624999385482941, 1.302750673588581876 ) ) ;
#10183=EDGE_LOOP ( 'NONE', ( #2454, #1788, #7754, #1294 ) ) ;
#10186=CARTESIAN_POINT ( 'NONE',  ( -1.728529299398585906, -5.253648441416169490, -1.450401466387756244 ) ) ;
#10187=CARTESIAN_POINT ( 'NONE',  ( 4.786228327491940187E-16, -1.940624999385482718, 2.605501347177161087 ) ) ;
#10189=CARTESIAN_POINT ( 'NONE',  ( -2.500000000000000000, -0.3937499987709658922, 0.000000000000000000 ) ) ;
#10193=CARTESIAN_POINT ( 'NONE',  ( -2.500000000000000000, -3.093749998770965348, 0.000000000000000000 ) ) ;
#10195=CARTESIAN_POINT ( 'NONE',  ( -2.500000000000000000, -2.643749998770965615, 0.000000000000000000 ) ) ;
#10197=VERTEX_POINT ( 'NONE', #5991 ) ;
#10198=CARTESIAN_POINT ( 'NONE',  ( -0.6698729810778105698, -4.351346188203299548, 2.499999999999997780 ) ) ;
#10199=CARTESIAN_POINT ( 'NONE',  ( -1.595409442497313560E-16, -1.153124999385483074, -2.605501347177161087 ) ) ;
#10207=ORIENTED_EDGE ( 'NONE', *, *, #8993, .F. ) ;
#10208=CARTESIAN_POINT ( 'NONE',  ( -2.499999999999999556, -3.112499999999999822, 1.443375672974065882 ) ) ;
#10211=CARTESIAN_POINT ( 'NONE',  ( 4.786228327491941173E-16, -1.490624999385482985, 2.605501347177161087 ) ) ;
#10214=ORIENTED_EDGE ( 'NONE', *, *, #8907, .T. ) ;
#10218=LINE ( 'NONE', #4555, #2229 ) ;
#10221=CARTESIAN_POINT ( 'NONE',  ( -2.256430356250000102, -0.1781249993854829572, -1.302750673588580321 ) ) ;
#10224=CARTESIAN_POINT ( 'NONE',  ( 2.256430356250000546, -1.303124999385482985, 1.302750673588579877 ) ) ;
#10234=CARTESIAN_POINT ( 'NONE',  ( -1.595409442497313560E-16, -3.515624999385482674, -2.605501347177161087 ) ) ;
#10235=VERTEX_POINT ( 'NONE', #4270 ) ;
#10239=CARTESIAN_POINT ( 'NONE',  ( 0.000000000000000000, 0.000000000000000000, -2.500000000000000000 ) ) ;
#10240=CARTESIAN_POINT ( 'NONE',  ( 2.256430356249999658, -0.4406249993854829961, -1.302750673588581432 ) ) ;
#10246=CARTESIAN_POINT ( 'NONE',  ( 2.500000000000000444, -2.456249998770965615, 1.443375672974063439 ) ) ;
#10253=CARTESIAN_POINT ( 'NONE',  ( -2.256430356249999214, -1.003124999385482718, 1.302750673588581876 ) ) ;
#10255=EDGE_CURVE ( 'NONE', #5851, #2954, #6936, .T. ) ;
#10260=ORIENTED_EDGE ( 'NONE', *, *, #6453, .F. ) ;
#10265=CARTESIAN_POINT ( 'NONE',  ( 2.500000000000000444, -4.762499999999999289, 1.443375672974063439 ) ) ;
#10267=CARTESIAN_POINT ( 'NONE',  ( 2.256430356250000102, -0.3656249993854829294, -2.763330213280484622E-16 ) ) ;
#10272=DIRECTION ( 'NONE',  ( 0.08704561088320923734, 0.9949358851208914833, 0.05025580687519627665 ) ) ;
#10275=CARTESIAN_POINT ( 'NONE',  ( 2.256430356249999658, -4.828124999385482674, -1.302750673588581432 ) ) ;
#10279=CARTESIAN_POINT ( 'NONE',  ( 1.128215178124999607, -2.090624999385482852, -1.954126010382871259 ) ) ;
#10280=( BOUNDED_CURVE ( )  B_SPLINE_CURVE ( 2, ( #7045, #10198, #7724, #7098, #5322, #3184, #10303, #4528, #6155 ),
 .UNSPECIFIED., .F., .T. ) 
 B_SPLINE_CURVE_WITH_KNOTS ( ( 3, 2, 2, 2, 3 ),
 ( 0.7291666666666667407, 0.7361111111111111605, 0.7500000000000000000, 0.7638888888888888395, 0.7708333333333333703 ),
 .UNSPECIFIED. ) 
 CURVE ( )  GEOMETRIC_REPRESENTATION_ITEM ( )  RATIONAL_B_SPLINE_CURVE ( ( 0.9330127018922192983, 0.9330127018922198534, 1.000000000000000000, 0.8660254037844387076, 1.000000000000000000, 0.8660254037844387076, 1.000000000000000000, 0.9330127018922187432, 0.9330127018922192983 ) ) 
 REPRESENTATION_ITEM ( '' )  );
#10288=CARTESIAN_POINT ( 'NONE',  ( -2.256430356250000102, -3.403124999385482408, 0.000000000000000000 ) ) ;
#10290=EDGE_CURVE ( 'NONE', #10048, #1242, #3270, .T. ) ;
#10294=CARTESIAN_POINT ( 'NONE',  ( 2.256430356250000102, -0.4781249993854829183, -2.763330213280484622E-16 ) ) ;
#10297=CARTESIAN_POINT ( 'NONE',  ( -1.767625397874844694E-16, -2.756249998770965437, -2.886751345948128655 ) ) ;
#10299=EDGE_CURVE ( 'NONE', #4436, #5524, #7324, .T. ) ;
#10303=CARTESIAN_POINT ( 'NONE',  ( -1.250000000000000222, -4.518749998770965171, -2.165063509461096825 ) ) ;
#10304=CARTESIAN_POINT ( 'NONE',  ( 4.786228327491941173E-16, -2.278124999385482852, 2.605501347177161087 ) ) ;
#10311=CARTESIAN_POINT ( 'NONE',  ( 1.250000000000001110, -2.999999999999999556, 2.165063509461096380 ) ) ;
#10315=CARTESIAN_POINT ( 'NONE',  ( -2.256430356250000102, -3.890624999385482674, -1.302750673588580321 ) ) ;
#10323=CARTESIAN_POINT ( 'NONE',  ( 3.061616997868383141E-16, 0.000000000000000000, 2.500000000000000000 ) ) ;
#10324=AXIS2_PLACEMENT_3D ( 'NONE', #9809, #3423, #4172 ) ;
#10325=CARTESIAN_POINT ( 'NONE',  ( -2.256430356250000102, -2.878124999385482941, -1.302750673588580321 ) ) ;
#10327=EDGE_LOOP ( 'NONE', ( #6859, #970, #2513, #8854 ) ) ;
#10329=CARTESIAN_POINT ( 'NONE',  ( -2.256430356250000102, -1.078124999385482896, -1.302750673588580321 ) ) ;
#10331=( LENGTH_UNIT ( ) NAMED_UNIT ( * ) SI_UNIT ( .MILLI., .METRE. ) );
#10332=CARTESIAN_POINT ( 'NONE',  ( 0.000000000000000000, 0.000000000000000000, 0.000000000000000000 ) ) ;
#10334=CARTESIAN_POINT ( 'NONE',  ( 9.877377282685029372E-16, -3.431249998770965259, 2.500000000000000000 ) ) ;
#10335=( GEOMETRIC_REPRESENTATION_CONTEXT ( 3 ) GLOBAL_UNCERTAINTY_ASSIGNED_CONTEXT ( ( #7690 ) ) GLOBAL_UNIT_ASSIGNED_CONTEXT ( ( #1042, #9730, #8950 ) ) REPRESENTATION_CONTEXT ( 'NONE', 'WORKASPACE' ) );
#10336=ORIENTED_EDGE ( 'NONE', *, *, #4623, .T. ) ;
#10340=CARTESIAN_POINT ( 'NONE',  ( 2.256430356250000546, -4.115624999385482319, 1.302750673588579877 ) ) ;
#10341=CARTESIAN_POINT ( 'NONE',  ( 0.6698729810778025762, -5.211153809338632037, 2.500000000000002665 ) ) ;
#10344=CARTESIAN_POINT ( 'NONE',  ( -3.486133158594716510E-16, -1.012499999999999956, -2.500000000000000000 ) ) ;
#10345=AXIS2_PLACEMENT_3D ( 'NONE', #9982, #3817, #7566 ) ;
#10346=CARTESIAN_POINT ( 'NONE',  ( -1.128215178125000273, -4.378124999385482496, -1.954126010382871259 ) ) ;
#10351=CARTESIAN_POINT ( 'NONE',  ( 1.250000000000001110, -1.143749998770965837, 2.165063509461096380 ) ) ;
#10355=CARTESIAN_POINT ( 'NONE',  ( -2.256430356249999214, -5.053124999385482319, 1.302750673588581876 ) ) ;
#10361=CARTESIAN_POINT ( 'NONE',  ( 0.6698729810778087934, -1.876346188203300347, -2.499999999999999112 ) ) ;
#10365=ORIENTED_EDGE ( 'NONE', *, *, #4409, .F. ) ;
#10388=COLOUR_RGB('Sky Blue',0.24,0.69,0.87);
#10389=FILL_AREA_STYLE_COLOUR('',#10388);
#10390=FILL_AREA_STYLE('',(#10389));
#10391=SURFACE_STYLE_FILL_AREA(#10390);
#10392=SURFACE_SIDE_STYLE('',(#10391));
#10393=SURFACE_STYLE_USAGE(.BOTH.,#10392);
#10394=PRESENTATION_STYLE_ASSIGNMENT((#10393));
ENDSEC;
END-ISO-10303-21;
